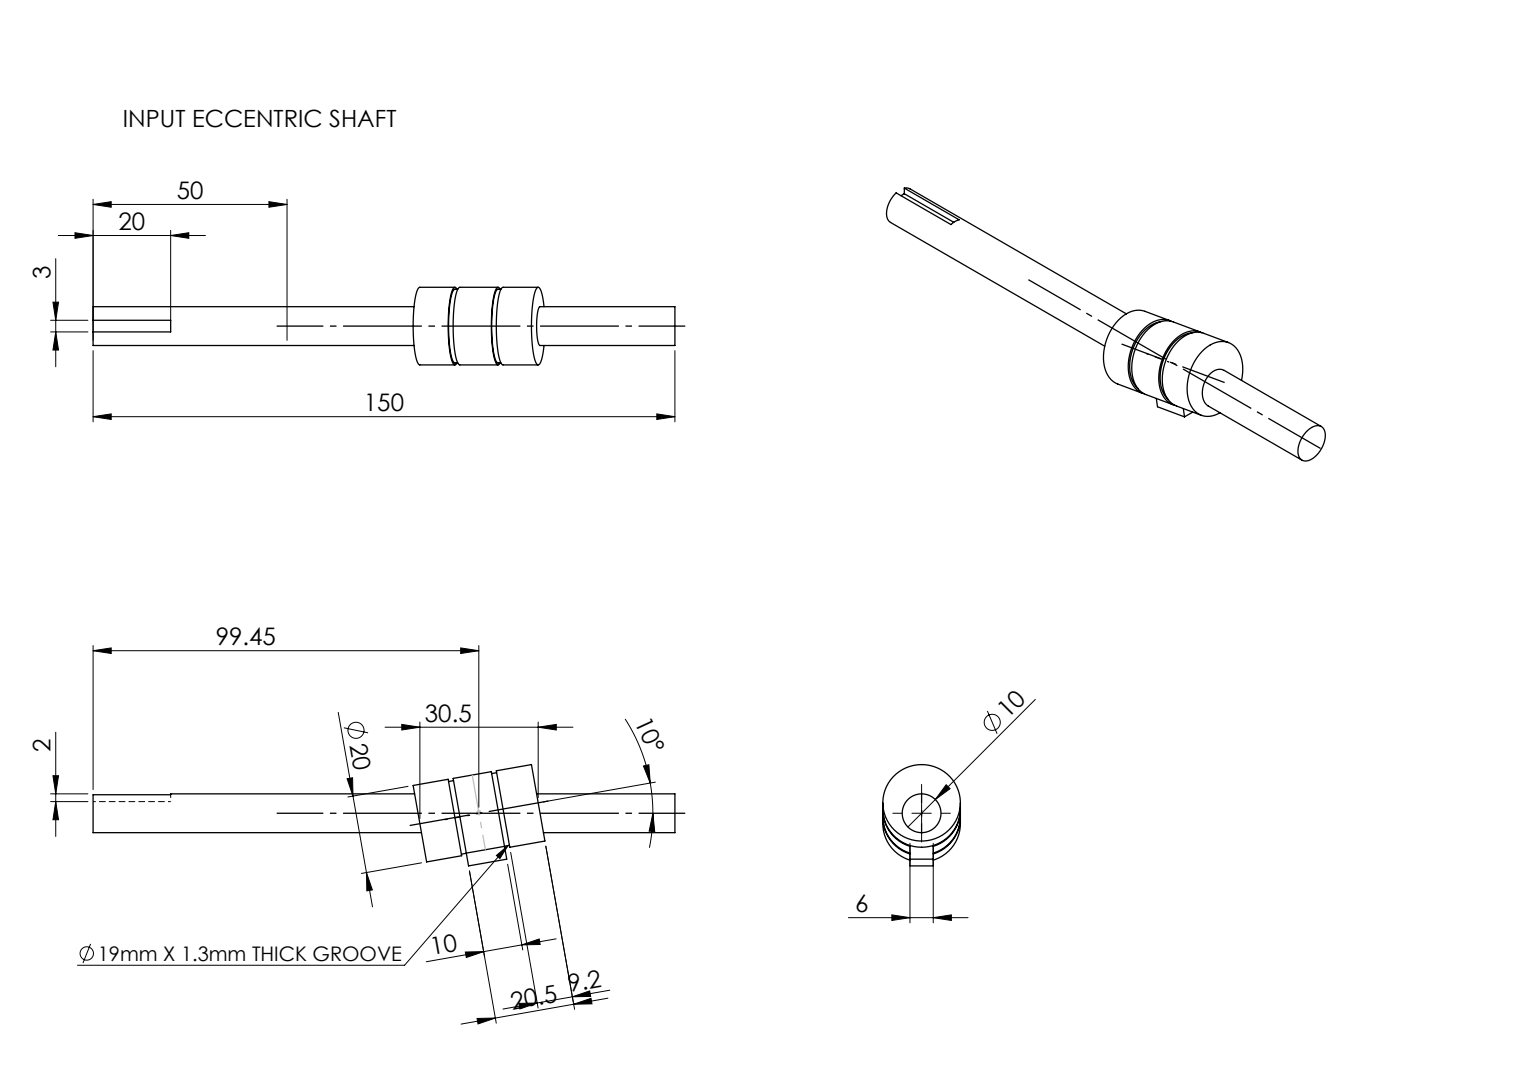
ISO-10303-21;
HEADER;
FILE_DESCRIPTION (('STEP AP214'),
    '1' );
FILE_NAME ('Input Eccentric Shaft.step',
    '2026-10-08T08:02:49',
    ( '' ),
    ( '' ),
    'SwSTEP 2.0',
    'SolidWorks 2026',
    '' );
FILE_SCHEMA (( 'AUTOMOTIVE_DESIGN' ));
ENDSEC;

DATA;
#16=CARTESIAN_POINT ( 'NONE',  ( 16.60577576646022635, -4.999999999999987566, 6.123233995736738672E-16 ) ) ;
#81=ORIENTED_EDGE ( 'NONE', *, *, #43581, .F. ) ;
#144=DIRECTION ( 'NONE',  ( 0.1736481776669314969, -0.9848077530122077983, 5.551115123125780853E-17 ) ) ;
#209=DIRECTION ( 'NONE',  ( -2.280301054154487250E-31, 0.000000000000000000, 1.000000000000000000 ) ) ;
#228=ORIENTED_EDGE ( 'NONE', *, *, #20971, .T. ) ;
#256=EDGE_CURVE ( 'NONE', #600, #12966, #42031, .T. ) ;
#273=FACE_OUTER_BOUND ( 'NONE', #5320, .T. ) ;
#336=MECHANICAL_DESIGN_GEOMETRIC_PRESENTATION_REPRESENTATION('',(#58375),#3336);
#521=AXIS2_PLACEMENT_3D ( 'NONE', #61352, #4959, #18467 ) ;
#546=CARTESIAN_POINT ( 'NONE',  ( 7.147292112312093160, -11.82536368408644911, -2.999999999999993339 ) ) ;
#552=ORIENTED_EDGE ( 'NONE', *, *, #15034, .T. ) ;
#600=VERTEX_POINT ( 'NONE', #1078 ) ;
#662=CARTESIAN_POINT ( 'NONE',  ( -2.700785417809989042, -13.56184546075576769, -3.000000000000003997 ) ) ;
#684=CIRCLE ( 'NONE', #45757, 9.499999999999996447 ) ;
#760=ORIENTED_EDGE ( 'NONE', *, *, #60258, .F. ) ;
#970=FACE_BOUND ( 'NONE', #13663, .T. ) ;
#1006=EDGE_CURVE ( 'NONE', #14410, #28664, #11050, .T. ) ;
#1078=CARTESIAN_POINT ( 'NONE',  ( -79.49999999999975842, 4.769696007084731626, 1.500000000000002220 ) ) ;
#1209=EDGE_CURVE ( 'NONE', #37522, #55939, #6365, .T. ) ;
#1224=CARTESIAN_POINT ( 'NONE',  ( -99.49999999999975842, -9.382821356248120971E-15, -1.500000000000001554 ) ) ;
#1342=LINE ( 'NONE', #2271, #20424 ) ;
#1460=DIRECTION ( 'NONE',  ( -0.1736481776669314137, 0.9848077530122079093, -5.551115123125779004E-17 ) ) ;
#1495=DIRECTION ( 'NONE',  ( -0.1736481776669314137, 0.9848077530122077983, -5.551115123125779004E-17 ) ) ;
#1496=ORIENTED_EDGE ( 'NONE', *, *, #49753, .T. ) ;
#1702=DIRECTION ( 'NONE',  ( 0.1736481776669314969, -0.9848077530122077983, 5.551115123125780853E-17 ) ) ;
#1775=DIRECTION ( 'NONE',  ( -0.9848077530122080203, -0.1736481776669315524, 2.220446049250313574E-16 ) ) ;
#1945=CYLINDRICAL_SURFACE ( 'NONE', #29493, 5.000000000000000000 ) ;
#2107=ORIENTED_EDGE ( 'NONE', *, *, #50234, .F. ) ;
#2130=CARTESIAN_POINT ( 'NONE',  ( -3.282060897439244229, -10.26526840094481052, -2.999999999999990674 ) ) ;
#2158=LINE ( 'NONE', #58242, #51760 ) ;
#2250=FACE_OUTER_BOUND ( 'NONE', #32718, .T. ) ;
#2271=CARTESIAN_POINT ( 'NONE',  ( -49.49999999999975842, -5.000000000000000000, 6.123233995736873765E-16 ) ) ;
#2292=ORIENTED_EDGE ( 'NONE', *, *, #4943, .T. ) ;
#2304=CIRCLE ( 'NONE', #10339, 10.00000000000000000 ) ;
#2335=PLANE ( 'NONE',  #54882 ) ;
#2340=LINE ( 'NONE', #46219, #9470 ) ;
#2383=DIRECTION ( 'NONE',  ( -1.000000000000000000, -1.836970198721027715E-16, 2.218671295934095703E-31 ) ) ;
#2463=CIRCLE ( 'NONE', #33486, 10.00000000000000711 ) ;
#2467=DIRECTION ( 'NONE',  ( 0.9848077530122080203, 0.1736481776669315524, -2.220446049250313574E-16 ) ) ;
#2493=DIRECTION ( 'NONE',  ( 4.437342591868191405E-31, -1.000000000000000000, -4.551914400963141816E-15 ) ) ;
#2607=ORIENTED_EDGE ( 'NONE', *, *, #38979, .F. ) ;
#2638=CARTESIAN_POINT ( 'NONE',  ( 7.147292112312088719, -11.82536368408648286, 3.000000000000017764 ) ) ;
#2691=VERTEX_POINT ( 'NONE', #5356 ) ;
#2704=CARTESIAN_POINT ( 'NONE',  ( -4.923482091946712380, -0.9563062221994939049, 3.000000000000061284 ) ) ;
#2772=ORIENTED_EDGE ( 'NONE', *, *, #49016, .T. ) ;
#2860=PRODUCT_DEFINITION_FORMATION_WITH_SPECIFIED_SOURCE ( 'ANY', '', #16779, .NOT_KNOWN. ) ;
#2948=DIRECTION ( 'NONE',  ( 2.280301054154487250E-31, 0.000000000000000000, -1.000000000000000000 ) ) ;
#3012=EDGE_LOOP ( 'NONE', ( #34469, #21920 ) ) ;
#3051=DIRECTION ( 'NONE',  ( 1.000000000000000000, 1.836970198721027962E-16, -2.033782021272921061E-31 ) ) ;
#3068=ADVANCED_FACE ( 'NONE', ( #57283 ), #53218, .F. ) ;
#3094=ADVANCED_FACE ( 'NONE', ( #273, #23485 ), #33217, .F. ) ;
#3103=EDGE_CURVE ( 'NONE', #36669, #44819, #10148, .T. ) ;
#3198=CIRCLE ( 'NONE', #15257, 5.000000000000000000 ) ;
#3247=ORIENTED_EDGE ( 'NONE', *, *, #59161, .T. ) ;
#3316=SURFACE_STYLE_FILL_AREA ( #40051 ) ;
#3325=VERTEX_POINT ( 'NONE', #34601 ) ;
#3336=( GEOMETRIC_REPRESENTATION_CONTEXT ( 3 ) GLOBAL_UNCERTAINTY_ASSIGNED_CONTEXT ( ( #22977 ) ) GLOBAL_UNIT_ASSIGNED_CONTEXT ( ( #55629, #50939, #7716 ) ) REPRESENTATION_CONTEXT ( 'NONE', 'WORKASPACE' ) );
#3383=DIRECTION ( 'NONE',  ( 0.1736481776669314969, -0.9848077530122079093, -4.496403249731880833E-15 ) ) ;
#3463=ORIENTED_EDGE ( 'NONE', *, *, #44142, .T. ) ;
#3467=CARTESIAN_POINT ( 'NONE',  ( -16.60577576646023701, 5.000000000000008882, -10.00000000000000711 ) ) ;
#3542=VECTOR ( 'NONE', #6303, 1000.000000000000114 ) ;
#3667=EDGE_CURVE ( 'NONE', #55095, #36276, #45940, .T. ) ;
#3711=EDGE_LOOP ( 'NONE', ( #32062, #21018 ) ) ;
#3726=ORIENTED_EDGE ( 'NONE', *, *, #22675, .T. ) ;
#3756=LINE ( 'NONE', #37313, #23956 ) ;
#3759=CARTESIAN_POINT ( 'NONE',  ( 0.000000000000000000, 0.000000000000000000, 0.000000000000000000 ) ) ;
#4057=EDGE_LOOP ( 'NONE', ( #59854, #35436, #34264, #58108, #27155 ) ) ;
#4066=EDGE_CURVE ( 'NONE', #5305, #44819, #39472, .T. ) ;
#4310=VECTOR ( 'NONE', #6048, 1000.000000000000000 ) ;
#4540=CYLINDRICAL_SURFACE ( 'NONE', #31521, 5.000000000000000000 ) ;
#4556=CARTESIAN_POINT ( 'NONE',  ( -6.573139779782565029, 8.399367431416496999, 5.684374357154926636E-14 ) ) ;
#4569=CARTESIAN_POINT ( 'NONE',  ( -16.60577576646023346, 5.000000000000006217, 4.095239503579248533E-30 ) ) ;
#4744=UNCERTAINTY_MEASURE_WITH_UNIT (LENGTH_MEASURE( 1.000000000000000082E-05 ), #37630, 'distance_accuracy_value', 'NONE');
#4762=DIRECTION ( 'NONE',  ( 0.9848077530122080203, 0.1736481776669314692, -5.551115123125783935E-17 ) ) ;
#4915=PLANE ( 'NONE',  #47230 ) ;
#4939=ORIENTED_EDGE ( 'NONE', *, *, #56201, .T. ) ;
#4943=EDGE_CURVE ( 'NONE', #55095, #58934, #3756, .T. ) ;
#4959=DIRECTION ( 'NONE',  ( 0.9848077530122080203, 0.1736481776669314692, -5.551115123125783935E-17 ) ) ;
#4976=DIRECTION ( 'NONE',  ( 0.1736481776669316079, -0.9848077530122079093, -5.551115123125822145E-17 ) ) ;
#5037=DIRECTION ( 'NONE',  ( -0.9848077530122079093, -0.1736481776669316357, -2.245658157333249735E-31 ) ) ;
#5054=DIRECTION ( 'NONE',  ( 0.000000000000000000, -1.000000000000000000, 0.000000000000000000 ) ) ;
#5130=CARTESIAN_POINT ( 'NONE',  ( 6.189768672337906175, 1.091423221261470733, -2.362915713819767774E-16 ) ) ;
#5234=VERTEX_POINT ( 'NONE', #12508 ) ;
#5274=ADVANCED_FACE ( 'NONE', ( #22206 ), #13427, .T. ) ;
#5305=VERTEX_POINT ( 'NONE', #28127 ) ;
#5320=EDGE_LOOP ( 'NONE', ( #35865, #19753 ) ) ;
#5356=CARTESIAN_POINT ( 'NONE',  ( 7.839426360173757047, -8.264250432354510068, 2.910643653149724807E-16 ) ) ;
#5414=DIRECTION ( 'NONE',  ( -0.1736481776669316357, 0.9848077530122079093, -5.551115123125819680E-17 ) ) ;
#5426=CARTESIAN_POINT ( 'NONE',  ( -15.25000000000000711, -2.688986455804108555, -9.952330921218299798E-16 ) ) ;
#5445=DIRECTION ( 'NONE',  ( 0.1736481776669314414, -0.9848077530122079093, 5.551115123125779621E-17 ) ) ;
#5497=EDGE_CURVE ( 'NONE', #2691, #3325, #18968, .T. ) ;
#5596=DIRECTION ( 'NONE',  ( -2.341930812374879235E-31, 1.110223024625156540E-16, 1.000000000000000000 ) ) ;
#5608=EDGE_CURVE ( 'NONE', #6174, #52714, #38324, .T. ) ;
#5613=DIRECTION ( 'NONE',  ( 1.000000000000000000, 1.836970198721029194E-16, -6.779273404243071298E-32 ) ) ;
#5645=DIRECTION ( 'NONE',  ( -2.280301054154487250E-31, 0.000000000000000000, 1.000000000000000000 ) ) ;
#5788=ORIENTED_EDGE ( 'NONE', *, *, #38677, .F. ) ;
#5814=VECTOR ( 'NONE', #17909, 1000.000000000000114 ) ;
#5835=ORIENTED_EDGE ( 'NONE', *, *, #15034, .F. ) ;
#5838=EDGE_CURVE ( 'NONE', #61564, #15021, #37028, .T. ) ;
#5904=CARTESIAN_POINT ( 'NONE',  ( 7.839426360173755270, -8.264250432354510068, 2.910643653149725793E-16 ) ) ;
#5997=EDGE_LOOP ( 'NONE', ( #8432, #36468, #1496, #44361, #29422 ) ) ;
#6020=CARTESIAN_POINT ( 'NONE',  ( 13.51351822333067965, 12.53706398592619209, -3.269553361041724978E-15 ) ) ;
#6048=DIRECTION ( 'NONE',  ( 1.000000000000000000, 1.836970198721027962E-16, -2.033782021272921061E-31 ) ) ;
#6061=ORIENTED_EDGE ( 'NONE', *, *, #8274, .T. ) ;
#6089=FACE_OUTER_BOUND ( 'NONE', #38846, .T. ) ;
#6119=EDGE_CURVE ( 'NONE', #24949, #36033, #38874, .T. ) ;
#6124=CARTESIAN_POINT ( 'NONE',  ( -79.49999999999975842, 5.000000000000006217, -1.500000000000003109 ) ) ;
#6174=VERTEX_POINT ( 'NONE', #36331 ) ;
#6215=CIRCLE ( 'NONE', #55238, 9.500000000000000000 ) ;
#6238=CARTESIAN_POINT ( 'NONE',  ( -4.482327238996802521, -10.94462134745707793, 2.754595595722048466E-16 ) ) ;
#6266=CIRCLE ( 'NONE', #17360, 10.00000000000000711 ) ;
#6303=DIRECTION ( 'NONE',  ( 0.9848077530122079093, 0.1736481776669314414, -5.551115123125783935E-17 ) ) ;
#6320=FACE_OUTER_BOUND ( 'NONE', #15017, .T. ) ;
#6363=EDGE_LOOP ( 'NONE', ( #27773, #60605, #46866, #11752 ) ) ;
#6365=( BOUNDED_CURVE ( )  B_SPLINE_CURVE ( 3, ( #9106, #3467, #14445, #61399 ),
 .UNSPECIFIED., .F., .F. ) 
 B_SPLINE_CURVE_WITH_KNOTS ( ( 4, 4 ),
 ( 3.141592653589793116, 6.283185307179586232 ),
 .UNSPECIFIED. ) 
 CURVE ( )  GEOMETRIC_REPRESENTATION_ITEM ( )  RATIONAL_B_SPLINE_CURVE ( ( 1.000000000000000000, 0.3333333333333333703, 0.3333333333333333703, 1.000000000000000000 ) ) 
 REPRESENTATION_ITEM ( '' )  );
#6400=VECTOR ( 'NONE', #40749, 1000.000000000000114 ) ;
#6421=AXIS2_PLACEMENT_3D ( 'NONE', #54757, #11891, #30970 ) ;
#6556=ORIENTED_EDGE ( 'NONE', *, *, #31470, .T. ) ;
#6626=CIRCLE ( 'NONE', #41706, 10.00000000000000711 ) ;
#6656=CARTESIAN_POINT ( 'NONE',  ( -15.25000000000000711, -2.688986455804108555, -9.952330921218299798E-16 ) ) ;
#6755=ORIENTED_EDGE ( 'NONE', *, *, #47460, .F. ) ;
#6883=DIRECTION ( 'NONE',  ( 0.9848077530122079093, 0.1736481776669314414, -5.551115123125783935E-17 ) ) ;
#6909=LINE ( 'NONE', #59544, #31718 ) ;
#6946=EDGE_LOOP ( 'NONE', ( #22828, #2607, #48957, #16108 ) ) ;
#7136=CARTESIAN_POINT ( 'NONE',  ( -99.49999999999975842, 2.999999999999993339, -1.278713541334263340E-16 ) ) ;
#7167=ORIENTED_EDGE ( 'NONE', *, *, #3667, .T. ) ;
#7246=EDGE_LOOP ( 'NONE', ( #40911, #30741 ) ) ;
#7323=EDGE_CURVE ( 'NONE', #15612, #55623, #24534, .T. ) ;
#7388=EDGE_LOOP ( 'NONE', ( #37494, #6556, #11509, #54224 ) ) ;
#7627=ADVANCED_FACE ( 'NONE', ( #34701, #15596 ), #40653, .F. ) ;
#7716=( NAMED_UNIT ( * ) SI_UNIT ( $, .STERADIAN. ) SOLID_ANGLE_UNIT ( ) );
#7789=VERTEX_POINT ( 'NONE', #60322 ) ;
#7823=AXIS2_PLACEMENT_3D ( 'NONE', #42228, #55976, #37524 ) ;
#7872=EDGE_LOOP ( 'NONE', ( #48131, #29211, #57257, #43270 ) ) ;
#7987=EDGE_CURVE ( 'NONE', #21914, #24949, #48711, .T. ) ;
#8086=DIRECTION ( 'NONE',  ( 0.1736481776669314137, -0.9848077530122077983, 9.436895709313830594E-16 ) ) ;
#8108=CARTESIAN_POINT ( 'NONE',  ( -14.84250595937556483, -4.999999999999993783, 6.123233995736803753E-16 ) ) ;
#8261=FACE_OUTER_BOUND ( 'NONE', #5997, .T. ) ;
#8274=EDGE_CURVE ( 'NONE', #37463, #37711, #43978, .T. ) ;
#8432=ORIENTED_EDGE ( 'NONE', *, *, #41048, .T. ) ;
#8496=DIRECTION ( 'NONE',  ( 0.000000000000000000, 1.000000000000000000, 0.000000000000000000 ) ) ;
#8549=ORIENTED_EDGE ( 'NONE', *, *, #57307, .F. ) ;
#8597=DIRECTION ( 'NONE',  ( 1.000000000000000000, 1.836970198721029194E-16, -6.779273404243071298E-32 ) ) ;
#8794=ORIENTED_EDGE ( 'NONE', *, *, #56127, .F. ) ;
#8921=EDGE_CURVE ( 'NONE', #37463, #45480, #43484, .T. ) ;
#8945=ORIENTED_EDGE ( 'NONE', *, *, #1006, .F. ) ;
#8994=FACE_OUTER_BOUND ( 'NONE', #13159, .T. ) ;
#9097=LINE ( 'NONE', #28206, #17938 ) ;
#9106=CARTESIAN_POINT ( 'NONE',  ( -16.60577576646023346, 5.000000000000006217, 4.095239503579248533E-30 ) ) ;
#9111=CARTESIAN_POINT ( 'NONE',  ( 3.259860905586184021, 10.22135424391044012, 4.719314477116953545E-16 ) ) ;
#9189=ADVANCED_FACE ( 'NONE', ( #2250 ), #1945, .T. ) ;
#9464=ORIENTED_EDGE ( 'NONE', *, *, #59161, .F. ) ;
#9470=VECTOR ( 'NONE', #55576, 1000.000000000000114 ) ;
#9517=DIRECTION ( 'NONE',  ( 0.9848077530122080203, 0.1736481776669315524, -2.220446049250313574E-16 ) ) ;
#9697=CARTESIAN_POINT ( 'NONE',  ( -4.923482091946715045, -0.9563062221994793610, 5.749747411347113621E-14 ) ) ;
#9732=ORIENTED_EDGE ( 'NONE', *, *, #57586, .F. ) ;
#9743=ORIENTED_EDGE ( 'NONE', *, *, #57307, .T. ) ;
#9943=CARTESIAN_POINT ( 'NONE',  ( -79.49999999999975842, -5.510910596163058790E-15, 1.848892746611746419E-29 ) ) ;
#10032=LINE ( 'NONE', #1224, #50554 ) ;
#10040=ORIENTED_EDGE ( 'NONE', *, *, #25957, .F. ) ;
#10148=CIRCLE ( 'NONE', #37175, 9.499999999999996447 ) ;
#10339=AXIS2_PLACEMENT_3D ( 'NONE', #43193, #23755, #42890 ) ;
#10511=VECTOR ( 'NONE', #23069, 1000.000000000000000 ) ;
#10651=CARTESIAN_POINT ( 'NONE',  ( -99.50001199999974233, 5.000000000000003553, -1.500000000000008216 ) ) ;
#10767=DIRECTION ( 'NONE',  ( 1.000000000000000000, 1.836970198721027962E-16, -2.033782021272921061E-31 ) ) ;
#10802=PLANE ( 'NONE',  #13161 ) ;
#10824=CYLINDRICAL_SURFACE ( 'NONE', #48633, 5.000000000000000000 ) ;
#10920=ORIENTED_EDGE ( 'NONE', *, *, #56201, .F. ) ;
#11050=LINE ( 'NONE', #43650, #12094 ) ;
#11308=DIRECTION ( 'NONE',  ( 0.9848077530122079093, 0.1736481776669315802, -5.551115123125782086E-17 ) ) ;
#11337=ORIENTED_EDGE ( 'NONE', *, *, #53081, .F. ) ;
#11483=LINE ( 'NONE', #49377, #28508 ) ;
#11509=ORIENTED_EDGE ( 'NONE', *, *, #17141, .F. ) ;
#11621=VERTEX_POINT ( 'NONE', #13879 ) ;
#11625=CYLINDRICAL_SURFACE ( 'NONE', #47390, 9.500000000000000000 ) ;
#11673=( GEOMETRIC_REPRESENTATION_CONTEXT ( 3 ) GLOBAL_UNCERTAINTY_ASSIGNED_CONTEXT ( ( #4744 ) ) GLOBAL_UNIT_ASSIGNED_CONTEXT ( ( #37630, #51074, #32298 ) ) REPRESENTATION_CONTEXT ( 'NONE', 'WORKASPACE' ) );
#11752=ORIENTED_EDGE ( 'NONE', *, *, #1006, .T. ) ;
#11830=ADVANCED_FACE ( 'NONE', ( #36309 ), #22194, .F. ) ;
#11891=DIRECTION ( 'NONE',  ( 0.9848077530122080203, 0.1736481776669315524, -2.220446049250313574E-16 ) ) ;
#11971=AXIS2_PLACEMENT_3D ( 'NONE', #54925, #31133, #50241 ) ;
#12089=DIRECTION ( 'NONE',  ( -0.1736481776669314137, 0.9848077530122079093, -5.551115123125779004E-17 ) ) ;
#12094=VECTOR ( 'NONE', #48624, 1000.000000000000114 ) ;
#12147=CARTESIAN_POINT ( 'NONE',  ( -6.203732170862584994, -1.182048853166489222, 5.744326400484686099E-14 ) ) ;
#12196=LINE ( 'NONE', #7136, #22678 ) ;
#12222=ORIENTED_EDGE ( 'NONE', *, *, #41831, .T. ) ;
#12249=FACE_OUTER_BOUND ( 'NONE', #6946, .T. ) ;
#12439=LINE ( 'NONE', #2704, #10511 ) ;
#12454=ADVANCED_FACE ( 'NONE', ( #44944 ), #19585, .T. ) ;
#12464=EDGE_LOOP ( 'NONE', ( #16584, #53415 ) ) ;
#12508=CARTESIAN_POINT ( 'NONE',  ( 6.559176281257887098, -8.489993063321520594, 3.632288619156076459E-16 ) ) ;
#12583=DIRECTION ( 'NONE',  ( 0.9848077530122079093, 0.1736481776669315524, -5.551115123125781470E-17 ) ) ;
#12627=CIRCLE ( 'NONE', #32600, 10.00000000000000355 ) ;
#12840=ORIENTED_EDGE ( 'NONE', *, *, #43546, .F. ) ;
#12842=EDGE_CURVE ( 'NONE', #38501, #36669, #6909, .T. ) ;
#12897=SURFACE_STYLE_USAGE ( .BOTH. , #46107 ) ;
#12966=VERTEX_POINT ( 'NONE', #27278 ) ;
#13133=ORIENTED_EDGE ( 'NONE', *, *, #47160, .T. ) ;
#13159=EDGE_LOOP ( 'NONE', ( #46438, #10040, #35648, #40443 ) ) ;
#13161=AXIS2_PLACEMENT_3D ( 'NONE', #58376, #58684, #39316 ) ;
#13350=ORIENTED_EDGE ( 'NONE', *, *, #25260, .T. ) ;
#13403=CARTESIAN_POINT ( 'NONE',  ( -49.49999999999975842, 1.232595164407830946E-29, 1.078520768856852078E-29 ) ) ;
#13427=CYLINDRICAL_SURFACE ( 'NONE', #37981, 10.00000000000000711 ) ;
#13470=AXIS2_PLACEMENT_3D ( 'NONE', #34635, #44665, #1702 ) ;
#13663=EDGE_LOOP ( 'NONE', ( #48253, #13133 ) ) ;
#13690=CIRCLE ( 'NONE', #49659, 10.00000000000000711 ) ;
#13778=CARTESIAN_POINT ( 'NONE',  ( -99.49999999999975842, -5.000000000000009770, 6.123233995736898417E-16 ) ) ;
#13822=DIRECTION ( 'NONE',  ( 1.000000000000000000, 0.000000000000000000, 0.000000000000000000 ) ) ;
#13879=CARTESIAN_POINT ( 'NONE',  ( -3.282060897439242453, -10.26526840094480164, 3.000000000000015987 ) ) ;
#13914=DIRECTION ( 'NONE',  ( -0.1736481776669312471, 0.9848077530122077983, -5.551115123125779621E-17 ) ) ;
#14098=ORIENTED_EDGE ( 'NONE', *, *, #8274, .F. ) ;
#14410=VERTEX_POINT ( 'NONE', #60838 ) ;
#14445=CARTESIAN_POINT ( 'NONE',  ( -14.84250595937557549, -4.999999999999997335, -10.00000000000000711 ) ) ;
#14662=DIRECTION ( 'NONE',  ( -0.9848077530122079093, -0.1736481776669316079, 5.551115123125783935E-17 ) ) ;
#14677=AXIS2_PLACEMENT_3D ( 'NONE', #3759, #61387, #13822 ) ;
#14867=EDGE_CURVE ( 'NONE', #37711, #37128, #6626, .T. ) ;
#15017=EDGE_LOOP ( 'NONE', ( #23318, #49149 ) ) ;
#15021=VERTEX_POINT ( 'NONE', #2130 ) ;
#15034=EDGE_CURVE ( 'NONE', #35339, #16043, #12196, .T. ) ;
#15131=CARTESIAN_POINT ( 'NONE',  ( -4.923482091946717709, -0.9563062221994661494, -2.999999999999945377 ) ) ;
#15141=FACE_OUTER_BOUND ( 'NONE', #37722, .T. ) ;
#15166=AXIS2_PLACEMENT_3D ( 'NONE', #42617, #61677, #47614 ) ;
#15257=AXIS2_PLACEMENT_3D ( 'NONE', #41389, #55135, #44857 ) ;
#15277=DIRECTION ( 'NONE',  ( -0.9848077530122079093, -0.1736481776669316357, -2.245658157333249735E-31 ) ) ;
#15460=DIRECTION ( 'NONE',  ( 1.000000000000000000, 1.836970198721027715E-16, -2.218671295934095703E-31 ) ) ;
#15567=DIRECTION ( 'NONE',  ( 1.836970198721031906E-16, -1.000000000000000000, 1.110223024625156540E-16 ) ) ;
#15596=FACE_OUTER_BOUND ( 'NONE', #3711, .T. ) ;
#15612=VERTEX_POINT ( 'NONE', #37792 ) ;
#15683=ADVANCED_FACE ( 'NONE', ( #44335 ), #10802, .T. ) ;
#15707=( GEOMETRIC_REPRESENTATION_CONTEXT ( 3 ) GLOBAL_UNCERTAINTY_ASSIGNED_CONTEXT ( ( #28578 ) ) GLOBAL_UNIT_ASSIGNED_CONTEXT ( ( #40801, #36092, #26980 ) ) REPRESENTATION_CONTEXT ( 'NONE', 'WORKASPACE' ) );
#15771=DIRECTION ( 'NONE',  ( -0.9848077530122079093, -0.1736481776669315802, 1.387778780781445367E-17 ) ) ;
#15843=PLANE ( 'NONE',  #57644 ) ;
#15894=LINE ( 'NONE', #25582, #26913 ) ;
#16043=VERTEX_POINT ( 'NONE', #31288 ) ;
#16108=ORIENTED_EDGE ( 'NONE', *, *, #3103, .T. ) ;
#16222=LINE ( 'NONE', #19693, #35442 ) ;
#16226=ADVANCED_FACE ( 'NONE', ( #19984, #39098 ), #4915, .T. ) ;
#16257=DIRECTION ( 'NONE',  ( -2.280301054154487250E-31, 0.000000000000000000, 1.000000000000000000 ) ) ;
#16372=DIRECTION ( 'NONE',  ( 1.000000000000000000, 1.836970198721027962E-16, -2.033782021272921061E-31 ) ) ;
#16416=ORIENTED_EDGE ( 'NONE', *, *, #5497, .F. ) ;
#16584=ORIENTED_EDGE ( 'NONE', *, *, #37344, .T. ) ;
#16779=PRODUCT ( 'Input Eccentric Shaft', 'Input Eccentric Shaft', '', ( #21797 ) ) ;
#16838=FILL_AREA_STYLE_COLOUR ( '', #26379 ) ;
#16911=VECTOR ( 'NONE', #10767, 1000.000000000000000 ) ;
#16928=AXIS2_PLACEMENT_3D ( 'NONE', #43300, #5037, #5645 ) ;
#16977=EDGE_LOOP ( 'NONE', ( #16416, #21342 ) ) ;
#17137=EDGE_CURVE ( 'NONE', #51465, #6174, #57525, .T. ) ;
#17141=EDGE_CURVE ( 'NONE', #5234, #46104, #6215, .T. ) ;
#17186=DIRECTION ( 'NONE',  ( 0.1736481776669316079, -0.9848077530122079093, -5.551115123125822145E-17 ) ) ;
#17360=AXIS2_PLACEMENT_3D ( 'NONE', #6656, #27040, #35840 ) ;
#17530=AXIS2_PLACEMENT_3D ( 'NONE', #53533, #58538, #33538 ) ;
#17550=ORIENTED_EDGE ( 'NONE', *, *, #256, .T. ) ;
#17661=CARTESIAN_POINT ( 'NONE',  ( 6.189768672337906175, 1.091423221261470733, -2.362915713819767774E-16 ) ) ;
#17747=CIRCLE ( 'NONE', #31747, 9.500000000000000000 ) ;
#17909=DIRECTION ( 'NONE',  ( -0.9848077530122079093, -0.1736481776669314414, 5.551115123125783935E-17 ) ) ;
#17938=VECTOR ( 'NONE', #47322, 1000.000000000000000 ) ;
#18111=DIRECTION ( 'NONE',  ( 0.9848077530122080203, 0.1736481776669315524, -2.220446049250313574E-16 ) ) ;
#18143=ORIENTED_EDGE ( 'NONE', *, *, #29937, .T. ) ;
#18202=SHAPE_REPRESENTATION_RELATIONSHIP ( 'NONE' , 'NONE' ,  #27649, #51224 ) ;
#18205=CARTESIAN_POINT ( 'NONE',  ( -79.49999999999975842, 4.999999999999996447, 1.500000000000000444 ) ) ;
#18371=EDGE_LOOP ( 'NONE', ( #14098, #56883, #20608, #20746 ) ) ;
#18437=LINE ( 'NONE', #23134, #21997 ) ;
#18467=DIRECTION ( 'NONE',  ( -0.1736481776669312471, 0.9848077530122077983, -5.551115123125779621E-17 ) ) ;
#18610=VECTOR ( 'NONE', #39599, 1000.000000000000000 ) ;
#18652=EDGE_LOOP ( 'NONE', ( #48864, #5788 ) ) ;
#18852=CARTESIAN_POINT ( 'NONE',  ( 14.84250595937556660, 5.000000000000015099, 10.00000000000000711 ) ) ;
#18878=DIRECTION ( 'NONE',  ( -0.1736481776669316357, 0.9848077530122079093, 4.662936703425656681E-15 ) ) ;
#18968=CIRCLE ( 'NONE', #20962, 9.500000000000000000 ) ;
#19051=EDGE_LOOP ( 'NONE', ( #52943, #17550, #37320, #4939 ) ) ;
#19487=FACE_OUTER_BOUND ( 'NONE', #29462, .T. ) ;
#19523=FACE_OUTER_BOUND ( 'NONE', #27402, .T. ) ;
#19585=CYLINDRICAL_SURFACE ( 'NONE', #21802, 9.500000000000005329 ) ;
#19614=ORIENTED_EDGE ( 'NONE', *, *, #5838, .T. ) ;
#19665=CARTESIAN_POINT ( 'NONE',  ( 4.540110984502055302, 10.44709687487745065, 3.997669511110601399E-16 ) ) ;
#19693=CARTESIAN_POINT ( 'NONE',  ( 4.924595438175360940, 0.7801755544698492084, -2.999999999999945821 ) ) ;
#19729=DIRECTION ( 'NONE',  ( -2.341930812374879235E-31, 1.110223024625156540E-16, 1.000000000000000000 ) ) ;
#19753=ORIENTED_EDGE ( 'NONE', *, *, #20975, .T. ) ;
#19815=AXIS2_PLACEMENT_3D ( 'NONE', #22245, #28781, #61657 ) ;
#19921=PRODUCT_DEFINITION_SHAPE ( 'NONE', 'NONE',  #43635 ) ;
#19984=FACE_OUTER_BOUND ( 'NONE', #39897, .T. ) ;
#20216=CIRCLE ( 'NONE', #45267, 9.500000000000000000 ) ;
#20360=CARTESIAN_POINT ( 'NONE',  ( -2.700785417809989042, -13.56184546075576769, -3.000000000000003997 ) ) ;
#20424=VECTOR ( 'NONE', #20479, 1000.000000000000000 ) ;
#20479=DIRECTION ( 'NONE',  ( 1.000000000000000000, 1.836970198721027962E-16, -2.033782021272921061E-31 ) ) ;
#20608=ORIENTED_EDGE ( 'NONE', *, *, #57586, .T. ) ;
#20692=PLANE ( 'NONE',  #32932 ) ;
#20746=ORIENTED_EDGE ( 'NONE', *, *, #14867, .F. ) ;
#20789=CIRCLE ( 'NONE', #19815, 5.000000000000000000 ) ;
#20962=AXIS2_PLACEMENT_3D ( 'NONE', #17661, #51456, #27058 ) ;
#20971=EDGE_CURVE ( 'NONE', #24192, #11621, #2463, .T. ) ;
#20975=EDGE_CURVE ( 'NONE', #36033, #24949, #47475, .T. ) ;
#21018=ORIENTED_EDGE ( 'NONE', *, *, #22675, .F. ) ;
#21022=VECTOR ( 'NONE', #56389, 1000.000000000000000 ) ;
#21086=CARTESIAN_POINT ( 'NONE',  ( -99.49999999999975842, -9.057560704502469641E-15, 1.500000000000000888 ) ) ;
#21342=ORIENTED_EDGE ( 'NONE', *, *, #30352, .F. ) ;
#21797=PRODUCT_CONTEXT ( 'NONE', #44793, 'mechanical' ) ;
#21802=AXIS2_PLACEMENT_3D ( 'NONE', #53072, #48383, #5445 ) ;
#21914=VERTEX_POINT ( 'NONE', #39550 ) ;
#21920=ORIENTED_EDGE ( 'NONE', *, *, #17137, .T. ) ;
#21942=LINE ( 'NONE', #41080, #56942 ) ;
#21997=VECTOR ( 'NONE', #3383, 1000.000000000000000 ) ;
#22001=ORIENTED_EDGE ( 'NONE', *, *, #53081, .T. ) ;
#22083=FACE_OUTER_BOUND ( 'NONE', #12464, .T. ) ;
#22179=EDGE_CURVE ( 'NONE', #2691, #5234, #33851, .T. ) ;
#22194=PLANE ( 'NONE',  #50757 ) ;
#22206=FACE_OUTER_BOUND ( 'NONE', #33124, .T. ) ;
#22236=CARTESIAN_POINT ( 'NONE',  ( 6.566016632731837888, -8.528786624275497275, -2.999999999999986677 ) ) ;
#22245=CARTESIAN_POINT ( 'NONE',  ( -99.49999999999975842, -9.184850993605117179E-15, 3.081487911019577365E-29 ) ) ;
#22527=CARTESIAN_POINT ( 'NONE',  ( -14.84250595937557016, -4.999999999999995559, 10.00000000000000711 ) ) ;
#22583=AXIS2_PLACEMENT_3D ( 'NONE', #47715, #4762, #13914 ) ;
#22591=FILL_AREA_STYLE ('',( #27590 ) ) ;
#22675=EDGE_CURVE ( 'NONE', #44582, #21914, #25945, .T. ) ;
#22678=VECTOR ( 'NONE', #16257, 1000.000000000000000 ) ;
#22828=ORIENTED_EDGE ( 'NONE', *, *, #4066, .F. ) ;
#22895=ORIENTED_EDGE ( 'NONE', *, *, #38677, .T. ) ;
#22977=UNCERTAINTY_MEASURE_WITH_UNIT (LENGTH_MEASURE( 1.000000000000000082E-05 ), #55629, 'distance_accuracy_value', 'NONE');
#23069=DIRECTION ( 'NONE',  ( 0.1736481776669314969, -0.9848077530122079093, -4.496403249731880833E-15 ) ) ;
#23134=CARTESIAN_POINT ( 'NONE',  ( 4.924595438175366269, 0.7801755544698232292, 3.000000000000058620 ) ) ;
#23309=CARTESIAN_POINT ( 'NONE',  ( -79.49999999999975842, -1.460391307983213802E-14, 1.540743955509788682E-30 ) ) ;
#23313=VECTOR ( 'NONE', #23816, 1000.000000000000114 ) ;
#23318=ORIENTED_EDGE ( 'NONE', *, *, #59797, .F. ) ;
#23485=FACE_BOUND ( 'NONE', #52507, .T. ) ;
#23556=CARTESIAN_POINT ( 'NONE',  ( -15.25000000000000711, -2.688986455804108555, -9.952330921218299798E-16 ) ) ;
#23585=ORIENTED_EDGE ( 'NONE', *, *, #43586, .T. ) ;
#23621=LINE ( 'NONE', #48353, #27892 ) ;
#23676=CARTESIAN_POINT ( 'NONE',  ( -49.49999999999975842, 1.232595164407830946E-29, 1.078520768856852078E-29 ) ) ;
#23755=DIRECTION ( 'NONE',  ( 0.9848077530122077983, 0.1736481776669316079, -1.387778780781445367E-17 ) ) ;
#23816=DIRECTION ( 'NONE',  ( -0.9848077530122079093, -0.1736481776669316079, 5.551115123125783935E-17 ) ) ;
#23872=DIRECTION ( 'NONE',  ( 0.9848077530122080203, 0.1736481776669314692, -5.551115123125783935E-17 ) ) ;
#23896=ORIENTED_EDGE ( 'NONE', *, *, #44390, .T. ) ;
#23956=VECTOR ( 'NONE', #31993, 1000.000000000000000 ) ;
#24192=VERTEX_POINT ( 'NONE', #40694 ) ;
#24450=CARTESIAN_POINT ( 'NONE',  ( 14.84250595937556483, 5.000000000000012434, -2.300655493813809945E-30 ) ) ;
#24534=CIRCLE ( 'NONE', #57551, 10.00000000000000000 ) ;
#24549=CIRCLE ( 'NONE', #37589, 10.00000000000000711 ) ;
#24552=DIRECTION ( 'NONE',  ( 0.1736481776669314137, -0.9848077530122077983, 5.551115123125779004E-17 ) ) ;
#24652=LINE ( 'NONE', #6124, #45372 ) ;
#24742=FACE_OUTER_BOUND ( 'NONE', #56323, .T. ) ;
#24805=VERTEX_POINT ( 'NONE', #29871 ) ;
#24815=PRODUCT_DEFINITION_CONTEXT ( 'detailed design', #50787, 'design' ) ;
#24874=FACE_OUTER_BOUND ( 'NONE', #49710, .T. ) ;
#24909=CIRCLE ( 'NONE', #40942, 5.000000000000000000 ) ;
#24949=VERTEX_POINT ( 'NONE', #37370 ) ;
#25042=VECTOR ( 'NONE', #55448, 1000.000000000000000 ) ;
#25051=FACE_OUTER_BOUND ( 'NONE', #51644, .T. ) ;
#25149=FACE_BOUND ( 'NONE', #16977, .T. ) ;
#25184=CARTESIAN_POINT ( 'NONE',  ( -49.49999999999975842, 5.000000000000000000, 1.078520768856852078E-29 ) ) ;
#25260=EDGE_CURVE ( 'NONE', #36276, #55939, #45783, .T. ) ;
#25365=ORIENTED_EDGE ( 'NONE', *, *, #31470, .F. ) ;
#25513=ORIENTED_EDGE ( 'NONE', *, *, #46681, .T. ) ;
#25582=CARTESIAN_POINT ( 'NONE',  ( 7.147292112312093160, -11.82536368408644911, -2.999999999999993339 ) ) ;
#25609=ORIENTED_EDGE ( 'NONE', *, *, #33336, .T. ) ;
#25711=DIRECTION ( 'NONE',  ( -0.1736481776669316357, 0.9848077530122079093, -5.551115123125819680E-17 ) ) ;
#25744=AXIS2_PLACEMENT_3D ( 'NONE', #9943, #61908, #52216 ) ;
#25790=AXIS2_PLACEMENT_3D ( 'NONE', #30396, #54498, #44234 ) ;
#25791=CYLINDRICAL_SURFACE ( 'NONE', #51920, 10.00000000000000711 ) ;
#25844=DIRECTION ( 'NONE',  ( 1.836970198721033632E-16, -1.000000000000000000, 0.000000000000000000 ) ) ;
#25945=CIRCLE ( 'NONE', #11971, 10.00000000000000711 ) ;
#25957=EDGE_CURVE ( 'NONE', #6174, #51465, #46220, .T. ) ;
#26200=CARTESIAN_POINT ( 'NONE',  ( -79.49999999999975842, -5.510910596163058790E-15, 1.848892746611746419E-29 ) ) ;
#26206=DIRECTION ( 'NONE',  ( 0.9848077530122079093, 0.1736481776669314137, -2.220446049250313081E-16 ) ) ;
#26236=CARTESIAN_POINT ( 'NONE',  ( -14.84250595937556483, -4.999999999999993783, 6.123233995736803753E-16 ) ) ;
#26379=COLOUR_RGB ( '', 0.40784314, 0.44705882, 0.49803922) ;
#26519=CARTESIAN_POINT ( 'NONE',  ( -15.25000000000000711, -2.688986455804108555, -9.952330921218299798E-16 ) ) ;
#26588=ADVANCED_FACE ( 'NONE', ( #53042 ), #37435, .T. ) ;
#26685=CIRCLE ( 'NONE', #32692, 5.000000000000000000 ) ;
#26801=( BOUNDED_CURVE ( )  B_SPLINE_CURVE ( 3, ( #8108, #22527, #33168, #27220 ),
 .UNSPECIFIED., .F., .F. ) 
 B_SPLINE_CURVE_WITH_KNOTS ( ( 4, 4 ),
 ( 0.000000000000000000, 3.141592653589793116 ),
 .UNSPECIFIED. ) 
 CURVE ( )  GEOMETRIC_REPRESENTATION_ITEM ( )  RATIONAL_B_SPLINE_CURVE ( ( 1.000000000000000000, 0.3333333333333333703, 0.3333333333333333703, 1.000000000000000000 ) ) 
 REPRESENTATION_ITEM ( '' )  );
#26913=VECTOR ( 'NONE', #35628, 1000.000000000000000 ) ;
#26949=CARTESIAN_POINT ( 'NONE',  ( -79.49999999999975842, 4.999999999999994671, 1.229372086083732569E-29 ) ) ;
#26980=( NAMED_UNIT ( * ) SI_UNIT ( $, .STERADIAN. ) SOLID_ANGLE_UNIT ( ) );
#27040=DIRECTION ( 'NONE',  ( 0.9848077530122080203, 0.1736481776669315247, -2.220446049250313081E-16 ) ) ;
#27058=DIRECTION ( 'NONE',  ( 0.1736481776669315247, -0.9848077530122079093, 5.551115123125782702E-17 ) ) ;
#27099=ADVANCED_FACE ( 'NONE', ( #50969 ), #36590, .T. ) ;
#27155=ORIENTED_EDGE ( 'NONE', *, *, #45156, .T. ) ;
#27202=ORIENTED_EDGE ( 'NONE', *, *, #41831, .F. ) ;
#27220=CARTESIAN_POINT ( 'NONE',  ( -16.60577576646023346, 5.000000000000006217, 4.095239503579248533E-30 ) ) ;
#27278=CARTESIAN_POINT ( 'NONE',  ( -79.49999999999975842, 2.999999999999996891, 1.500000000000000000 ) ) ;
#27285=CARTESIAN_POINT ( 'NONE',  ( -79.49999999999975842, 4.769696007084728961, -1.500000000000002887 ) ) ;
#27299=ORIENTED_EDGE ( 'NONE', *, *, #5608, .F. ) ;
#27402=EDGE_LOOP ( 'NONE', ( #28240, #228, #47775, #54695 ) ) ;
#27495=DIRECTION ( 'NONE',  ( 0.1736481776669315247, -0.9848077530122079093, 5.551115123125782702E-17 ) ) ;
#27499=CARTESIAN_POINT ( 'NONE',  ( -4.938558936750251149, -0.8708011863679817610, 8.896908036367455278E-17 ) ) ;
#27556=CYLINDRICAL_SURFACE ( 'NONE', #521, 10.00000000000000711 ) ;
#27590=FILL_AREA_STYLE_COLOUR ( '', #50682 ) ;
#27649=SHAPE_REPRESENTATION ( 'Input Eccentric Shaft', ( #14677 ), #15707 ) ;
#27725=LINE ( 'NONE', #52132, #30832 ) ;
#27759=VECTOR ( 'NONE', #47424, 1000.000000000000000 ) ;
#27773=ORIENTED_EDGE ( 'NONE', *, *, #45156, .F. ) ;
#27849=CIRCLE ( 'NONE', #25744, 5.000000000000000000 ) ;
#27857=EDGE_LOOP ( 'NONE', ( #552, #2772, #25513, #27202 ) ) ;
#27866=ADVANCED_FACE ( 'NONE', ( #19487 ), #28252, .F. ) ;
#27892=VECTOR ( 'NONE', #53341, 1000.000000000000114 ) ;
#28102=CYLINDRICAL_SURFACE ( 'NONE', #36371, 5.000000000000000000 ) ;
#28127=CARTESIAN_POINT ( 'NONE',  ( -4.554074483026735898, -10.53772250678246358, 5.913403440073379425E-14 ) ) ;
#28206=CARTESIAN_POINT ( 'NONE',  ( -2.700785417809989042, -13.56184546075576769, -3.000000000000003997 ) ) ;
#28240=ORIENTED_EDGE ( 'NONE', *, *, #44142, .F. ) ;
#28252=PLANE ( 'NONE',  #38892 ) ;
#28254=DIRECTION ( 'NONE',  ( -0.1736481776669312471, 0.9848077530122077983, -5.551115123125779621E-17 ) ) ;
#28434=ORIENTED_EDGE ( 'NONE', *, *, #30352, .T. ) ;
#28473=AXIS2_PLACEMENT_3D ( 'NONE', #41617, #32214, #17186 ) ;
#28508=VECTOR ( 'NONE', #44108, 1000.000000000000114 ) ;
#28578=UNCERTAINTY_MEASURE_WITH_UNIT (LENGTH_MEASURE( 1.000000000000000082E-05 ), #40801, 'distance_accuracy_value', 'NONE');
#28609=LINE ( 'NONE', #33342, #27759 ) ;
#28664=VERTEX_POINT ( 'NONE', #2638 ) ;
#28781=DIRECTION ( 'NONE',  ( -1.000000000000000000, -1.836970198721027715E-16, 2.218671295934095703E-31 ) ) ;
#28821=ADVANCED_FACE ( 'NONE', ( #44834 ), #20692, .T. ) ;
#28928=DIRECTION ( 'NONE',  ( 0.1736481776669315802, -0.9848077530122079093, 5.551115123125782702E-17 ) ) ;
#28929=ADVANCED_FACE ( 'NONE', ( #43930, #970 ), #33584, .F. ) ;
#29164=CARTESIAN_POINT ( 'NONE',  ( 6.566016632682842413, -8.528786624275486616, 3.000000000000020872 ) ) ;
#29211=ORIENTED_EDGE ( 'NONE', *, *, #43546, .T. ) ;
#29418=CARTESIAN_POINT ( 'NONE',  ( -99.50001199999974233, 5.000000000000001776, 1.500000000000000222 ) ) ;
#29422=ORIENTED_EDGE ( 'NONE', *, *, #256, .F. ) ;
#29462=EDGE_LOOP ( 'NONE', ( #23896, #8945, #34005, #22001 ) ) ;
#29493=AXIS2_PLACEMENT_3D ( 'NONE', #59265, #16372, #8496 ) ;
#29559=ADVANCED_FACE ( 'NONE', ( #24874 ), #25791, .T. ) ;
#29739=PLANE ( 'NONE',  #46560 ) ;
#29749=CARTESIAN_POINT ( 'NONE',  ( -7.853389858698435866, 8.173624800449486472, 5.691590806814991163E-14 ) ) ;
#29826=DIRECTION ( 'NONE',  ( 0.1736481776669314969, -0.9848077530122079093, -4.496403249731880833E-15 ) ) ;
#29871=CARTESIAN_POINT ( 'NONE',  ( -99.49999999999975842, 4.769696007084727185, 1.499999999999998446 ) ) ;
#29896=VECTOR ( 'NONE', #58220, 1000.000000000000000 ) ;
#29937=EDGE_CURVE ( 'NONE', #7789, #52714, #3198, .T. ) ;
#30038=CARTESIAN_POINT ( 'NONE',  ( 15.24999999999999289, 2.688986455804112996, 8.896908036367455278E-17 ) ) ;
#30186=LINE ( 'NONE', #25184, #4310 ) ;
#30228=DIRECTION ( 'NONE',  ( -1.000000000000000000, -1.836970198721033632E-16, 2.218671295934095703E-31 ) ) ;
#30352=EDGE_CURVE ( 'NONE', #3325, #2691, #20216, .T. ) ;
#30396=CARTESIAN_POINT ( 'NONE',  ( -4.923482091946715045, -0.9563062221994793610, 5.749747411347113621E-14 ) ) ;
#30464=LINE ( 'NONE', #21086, #18610 ) ;
#30472=DIRECTION ( 'NONE',  ( 0.9848077530122080203, 0.1736481776669314692, -5.551115123125783935E-17 ) ) ;
#30654=MECHANICAL_DESIGN_GEOMETRIC_PRESENTATION_REPRESENTATION('',(#49663),#11673);
#30741=ORIENTED_EDGE ( 'NONE', *, *, #48278, .F. ) ;
#30832=VECTOR ( 'NONE', #8597, 1000.000000000000000 ) ;
#30938=CARTESIAN_POINT ( 'NONE',  ( 14.84250595937556483, 5.000000000000015099, -10.00000000000000711 ) ) ;
#30970=DIRECTION ( 'NONE',  ( 0.1736481776669314137, -0.9848077530122077983, 5.551115123125779621E-17 ) ) ;
#31133=DIRECTION ( 'NONE',  ( 0.9848077530122080203, 0.1736481776669315247, -2.220446049250313081E-16 ) ) ;
#31245=CARTESIAN_POINT ( 'NONE',  ( 16.60577576646022635, -4.999999999999987566, 6.123233995736738672E-16 ) ) ;
#31288=CARTESIAN_POINT ( 'NONE',  ( -99.49999999999975842, 2.999999999999994671, 1.500000000000001554 ) ) ;
#31470=EDGE_CURVE ( 'NONE', #3325, #46104, #48460, .T. ) ;
#31517=CIRCLE ( 'NONE', #28473, 9.499999999999996447 ) ;
#31521=AXIS2_PLACEMENT_3D ( 'NONE', #23676, #33401, #52478 ) ;
#31624=LINE ( 'NONE', #60120, #6400 ) ;
#31718=VECTOR ( 'NONE', #12583, 1000.000000000000000 ) ;
#31747=AXIS2_PLACEMENT_3D ( 'NONE', #34492, #54175, #43917 ) ;
#31993=DIRECTION ( 'NONE',  ( 1.000000000000000000, 1.836970198721027962E-16, -2.033782021272921061E-31 ) ) ;
#32062=ORIENTED_EDGE ( 'NONE', *, *, #50356, .F. ) ;
#32214=DIRECTION ( 'NONE',  ( -0.9848077530122080203, -0.1736481776669315524, 2.220446049250313574E-16 ) ) ;
#32266=ADVANCED_FACE ( 'NONE', ( #12249 ), #11625, .T. ) ;
#32298=( NAMED_UNIT ( * ) SI_UNIT ( $, .STERADIAN. ) SOLID_ANGLE_UNIT ( ) );
#32370=ORIENTED_EDGE ( 'NONE', *, *, #4943, .F. ) ;
#32441=VERTEX_POINT ( 'NONE', #26949 ) ;
#32535=CARTESIAN_POINT ( 'NONE',  ( -15.25000000000000711, -2.688986455804108555, -9.952330921218299798E-16 ) ) ;
#32600=AXIS2_PLACEMENT_3D ( 'NONE', #47483, #43107, #144 ) ;
#32692=AXIS2_PLACEMENT_3D ( 'NONE', #26200, #2383, #59397 ) ;
#32718=EDGE_LOOP ( 'NONE', ( #45990, #25609, #52166, #27299 ) ) ;
#32727=DIRECTION ( 'NONE',  ( 0.9848077530122079093, 0.1736481776669315802, -5.551115123125782086E-17 ) ) ;
#32800=ORIENTED_EDGE ( 'NONE', *, *, #25260, .F. ) ;
#32818=ADVANCED_FACE ( 'NONE', ( #8994 ), #28102, .T. ) ;
#32932=AXIS2_PLACEMENT_3D ( 'NONE', #40755, #39831, #2493 ) ;
#33046=CARTESIAN_POINT ( 'NONE',  ( -4.938558936750251149, -0.8708011863679817610, 8.896908036367455278E-17 ) ) ;
#33124=EDGE_LOOP ( 'NONE', ( #58141, #3463, #61395, #19614 ) ) ;
#33168=CARTESIAN_POINT ( 'NONE',  ( -16.60577576646022990, 5.000000000000008882, 10.00000000000000711 ) ) ;
#33217=PLANE ( 'NONE',  #15166 ) ;
#33259=DIRECTION ( 'NONE',  ( 0.1736481776669315247, -0.9848077530122079093, 5.551115123125782702E-17 ) ) ;
#33336=EDGE_CURVE ( 'NONE', #51465, #7789, #1342, .T. ) ;
#33342=CARTESIAN_POINT ( 'NONE',  ( -79.49999999999975842, 2.999999999999996891, 1.500000000000000000 ) ) ;
#33401=DIRECTION ( 'NONE',  ( 1.000000000000000000, 1.836970198721027962E-16, -2.033782021272921061E-31 ) ) ;
#33486=AXIS2_PLACEMENT_3D ( 'NONE', #27499, #18111, #8086 ) ;
#33538=DIRECTION ( 'NONE',  ( 4.437342591868191405E-31, -1.000000000000000000, -4.551914400963141816E-15 ) ) ;
#33559=ADVANCED_FACE ( 'NONE', ( #52358 ), #42383, .T. ) ;
#33584=PLANE ( 'NONE',  #16928 ) ;
#33838=DIRECTION ( 'NONE',  ( 2.218671295934095703E-31, -1.000000000000000000, 1.110223024625156540E-16 ) ) ;
#33851=LINE ( 'NONE', #5904, #23313 ) ;
#33955=CARTESIAN_POINT ( 'NONE',  ( -99.49999999999975842, 4.769696007084730738, -1.500000000000008438 ) ) ;
#33979=DIRECTION ( 'NONE',  ( -0.1736481776669312471, 0.9848077530122077983, -5.551115123125779621E-17 ) ) ;
#34005=ORIENTED_EDGE ( 'NONE', *, *, #44839, .F. ) ;
#34179=CARTESIAN_POINT ( 'NONE',  ( 16.60577576646022990, -4.999999999999989342, 10.00000000000000711 ) ) ;
#34248=CYLINDRICAL_SURFACE ( 'NONE', #49616, 10.00000000000000711 ) ;
#34264=ORIENTED_EDGE ( 'NONE', *, *, #50707, .T. ) ;
#34266=CARTESIAN_POINT ( 'NONE',  ( -49.49999999999975842, 4.769696007084739620, 1.500000000000005329 ) ) ;
#34469=ORIENTED_EDGE ( 'NONE', *, *, #25957, .T. ) ;
#34492=CARTESIAN_POINT ( 'NONE',  ( 4.909518593422035337, 0.8656805902944597619, 8.896908036367455278E-17 ) ) ;
#34601=CARTESIAN_POINT ( 'NONE',  ( 4.540110984502054414, 10.44709687487745065, 3.997669511110601399E-16 ) ) ;
#34635=CARTESIAN_POINT ( 'NONE',  ( 6.189768672335216770, 1.091423221276722755, -1.945113688487589062E-17 ) ) ;
#34701=FACE_BOUND ( 'NONE', #18652, .T. ) ;
#34739=CARTESIAN_POINT ( 'NONE',  ( 15.24999999999999289, 2.688986455804112996, 8.896908036367455278E-17 ) ) ;
#34957=CARTESIAN_POINT ( 'NONE',  ( -99.49999999999975842, -9.184850993605117179E-15, 3.081487911019577365E-29 ) ) ;
#35339=VERTEX_POINT ( 'NONE', #39739 ) ;
#35436=ORIENTED_EDGE ( 'NONE', *, *, #51896, .F. ) ;
#35442=VECTOR ( 'NONE', #40064, 1000.000000000000000 ) ;
#35628=DIRECTION ( 'NONE',  ( 8.032841876251139751E-16, -4.551914400963141816E-15, 1.000000000000000000 ) ) ;
#35648=ORIENTED_EDGE ( 'NONE', *, *, #5608, .T. ) ;
#35840=DIRECTION ( 'NONE',  ( -0.1736481776669312471, 0.9848077530122077983, -5.551115123125779621E-17 ) ) ;
#35865=ORIENTED_EDGE ( 'NONE', *, *, #6119, .T. ) ;
#35885=CARTESIAN_POINT ( 'NONE',  ( 15.24999999999999289, 2.688986455804112996, 8.896908036367455278E-17 ) ) ;
#35955=PRESENTATION_STYLE_ASSIGNMENT (( #60327 ) ) ;
#36033=VERTEX_POINT ( 'NONE', #6238 ) ;
#36092=( NAMED_UNIT ( * ) PLANE_ANGLE_UNIT ( ) SI_UNIT ( $, .RADIAN. ) );
#36276=VERTEX_POINT ( 'NONE', #13778 ) ;
#36309=FACE_OUTER_BOUND ( 'NONE', #27857, .T. ) ;
#36331=CARTESIAN_POINT ( 'NONE',  ( 14.84250595937556483, 5.000000000000012434, -2.300655493813809945E-30 ) ) ;
#36371=AXIS2_PLACEMENT_3D ( 'NONE', #13403, #3051, #41303 ) ;
#36468=ORIENTED_EDGE ( 'NONE', *, *, #49696, .T. ) ;
#36590=CYLINDRICAL_SURFACE ( 'NONE', #7823, 9.500000000000005329 ) ;
#36669=VERTEX_POINT ( 'NONE', #4556 ) ;
#36808=ORIENTED_EDGE ( 'NONE', *, *, #50234, .T. ) ;
#36810=PLANE ( 'NONE',  #43805 ) ;
#36932=DIRECTION ( 'NONE',  ( 1.836970198721027962E-16, -1.000000000000000000, 1.069580750882383731E-61 ) ) ;
#36996=VECTOR ( 'NONE', #53002, 1000.000000000000000 ) ;
#37028=LINE ( 'NONE', #52007, #5814 ) ;
#37116=CARTESIAN_POINT ( 'NONE',  ( 16.60577576646022635, -4.999999999999987566, 6.123233995736738672E-16 ) ) ;
#37128=VERTEX_POINT ( 'NONE', #6020 ) ;
#37175=AXIS2_PLACEMENT_3D ( 'NONE', #9697, #47928, #4976 ) ;
#37313=CARTESIAN_POINT ( 'NONE',  ( -49.49999999999975842, 4.769696007084736067, -1.500000000000002220 ) ) ;
#37320=ORIENTED_EDGE ( 'NONE', *, *, #49016, .F. ) ;
#37344=EDGE_CURVE ( 'NONE', #37128, #37711, #13690, .T. ) ;
#37348=EDGE_LOOP ( 'NONE', ( #32800, #51309, #2292, #43294, #36808, #53375 ) ) ;
#37370=CARTESIAN_POINT ( 'NONE',  ( -7.955290792335435235, 8.751533712787090025, -2.059410264200305690E-15 ) ) ;
#37435=CYLINDRICAL_SURFACE ( 'NONE', #53820, 9.500000000000000000 ) ;
#37463=VERTEX_POINT ( 'NONE', #60665 ) ;
#37494=ORIENTED_EDGE ( 'NONE', *, *, #5497, .T. ) ;
#37522=VERTEX_POINT ( 'NONE', #4569 ) ;
#37524=DIRECTION ( 'NONE',  ( 0.1736481776669314414, -0.9848077530122079093, 5.551115123125779621E-17 ) ) ;
#37589=AXIS2_PLACEMENT_3D ( 'NONE', #33046, #9517, #24552 ) ;
#37630=( LENGTH_UNIT ( ) NAMED_UNIT ( * ) SI_UNIT ( .MILLI., .METRE. ) );
#37711=VERTEX_POINT ( 'NONE', #44391 ) ;
#37721=CYLINDRICAL_SURFACE ( 'NONE', #22583, 10.00000000000000711 ) ;
#37722=EDGE_LOOP ( 'NONE', ( #12840, #3726, #53778, #57855 ) ) ;
#37755=CARTESIAN_POINT ( 'NONE',  ( -6.203732170862584994, -1.182048853166489222, 5.744326400484686099E-14 ) ) ;
#37792=CARTESIAN_POINT ( 'NONE',  ( 3.173036816750036238, 10.71375812043179643, -2.686686273116197949E-15 ) ) ;
#37915=FACE_OUTER_BOUND ( 'NONE', #7872, .T. ) ;
#37981=AXIS2_PLACEMENT_3D ( 'NONE', #32535, #45720, #51614 ) ;
#38051=DIRECTION ( 'NONE',  ( -0.1736481776669312471, 0.9848077530122077983, -5.551115123125779621E-17 ) ) ;
#38324=LINE ( 'NONE', #38631, #36996 ) ;
#38501=VERTEX_POINT ( 'NONE', #29749 ) ;
#38631=CARTESIAN_POINT ( 'NONE',  ( -49.49999999999975842, 5.000000000000000000, 1.078520768856852078E-29 ) ) ;
#38668=LINE ( 'NONE', #34266, #16911 ) ;
#38677=EDGE_CURVE ( 'NONE', #55939, #37522, #26801, .T. ) ;
#38695=DIRECTION ( 'NONE',  ( -0.9848077530122077983, -0.1736481776669316079, 1.387778780781445367E-17 ) ) ;
#38846=EDGE_LOOP ( 'NONE', ( #5835, #3247, #7167, #61690, #10920 ) ) ;
#38874=CIRCLE ( 'NONE', #39864, 10.00000000000000711 ) ;
#38892=AXIS2_PLACEMENT_3D ( 'NONE', #662, #18878, #47365 ) ;
#38952=DIRECTION ( 'NONE',  ( 0.1736481776669315524, -0.9848077530122079093, 5.551115123125782702E-17 ) ) ;
#38979=EDGE_CURVE ( 'NONE', #38501, #5305, #684, .T. ) ;
#39098=FACE_BOUND ( 'NONE', #7246, .T. ) ;
#39316=DIRECTION ( 'NONE',  ( -1.836970198721033632E-16, 1.000000000000000000, 0.000000000000000000 ) ) ;
#39337=CARTESIAN_POINT ( 'NONE',  ( -16.98648177666931858, 7.159091074317976755, -1.550344604434408250E-15 ) ) ;
#39362=VECTOR ( 'NONE', #14662, 1000.000000000000114 ) ;
#39472=LINE ( 'NONE', #43247, #29896 ) ;
#39481=DIRECTION ( 'NONE',  ( -1.836970198721032153E-16, 1.000000000000000000, -1.110223024625156540E-16 ) ) ;
#39550=CARTESIAN_POINT ( 'NONE',  ( -16.98648177666932213, 7.159091074317976755, -1.550344604434408250E-15 ) ) ;
#39599=DIRECTION ( 'NONE',  ( -1.836970198721032153E-16, 1.000000000000000000, -1.110223024625156540E-16 ) ) ;
#39739=CARTESIAN_POINT ( 'NONE',  ( -99.49999999999975842, 2.999999999999992895, -1.500000000000000666 ) ) ;
#39831=DIRECTION ( 'NONE',  ( 7.985424459127866231E-16, -4.551914400963141816E-15, 1.000000000000000000 ) ) ;
#39864=AXIS2_PLACEMENT_3D ( 'NONE', #54459, #2467, #53842 ) ;
#39897=EDGE_LOOP ( 'NONE', ( #54927, #42327, #61704, #8794, #46135 ) ) ;
#39910=DIRECTION ( 'NONE',  ( 0.000000000000000000, 1.000000000000000000, 0.000000000000000000 ) ) ;
#39970=DIRECTION ( 'NONE',  ( 0.9848077530122079093, 0.1736481776669314414, -5.551115123125783935E-17 ) ) ;
#39974=DIRECTION ( 'NONE',  ( 1.000000000000000000, 1.836970198721027962E-16, -2.033782021272921061E-31 ) ) ;
#40051=FILL_AREA_STYLE ('',( #16838 ) ) ;
#40064=DIRECTION ( 'NONE',  ( 0.1736481776669314969, -0.9848077530122079093, -4.496403249731880833E-15 ) ) ;
#40443=ORIENTED_EDGE ( 'NONE', *, *, #29937, .F. ) ;
#40653=PLANE ( 'NONE',  #59536 ) ;
#40657=DIRECTION ( 'NONE',  ( 0.1736481776669316079, -0.9848077530122079093, -5.551115123125822145E-17 ) ) ;
#40694=CARTESIAN_POINT ( 'NONE',  ( -6.675040713419566174, 8.977276343754100552, -2.131574760800940707E-15 ) ) ;
#40749=DIRECTION ( 'NONE',  ( -0.9848077530122079093, -0.1736481776669314414, 5.551115123125783935E-17 ) ) ;
#40755=CARTESIAN_POINT ( 'NONE',  ( -4.923482091946712380, -0.9563062221994939049, 3.000000000000061284 ) ) ;
#40801=( LENGTH_UNIT ( ) NAMED_UNIT ( * ) SI_UNIT ( .MILLI., .METRE. ) );
#40911=ORIENTED_EDGE ( 'NONE', *, *, #3103, .F. ) ;
#40942=AXIS2_PLACEMENT_3D ( 'NONE', #43367, #15460, #39910 ) ;
#41048=EDGE_CURVE ( 'NONE', #600, #32441, #26685, .T. ) ;
#41080=CARTESIAN_POINT ( 'NONE',  ( -16.98648177666931858, 7.159091074317976755, -1.550344604434408250E-15 ) ) ;
#41200=DIRECTION ( 'NONE',  ( 1.000000000000000000, 1.836970198721027715E-16, 2.280301054154487250E-31 ) ) ;
#41303=DIRECTION ( 'NONE',  ( 0.000000000000000000, 1.000000000000000000, 0.000000000000000000 ) ) ;
#41317=CARTESIAN_POINT ( 'NONE',  ( -99.50001199999974233, 2.999999999999994671, 1.500000000000001554 ) ) ;
#41389=CARTESIAN_POINT ( 'NONE',  ( 50.50000000000024869, 1.836970198721029747E-14, -7.703719777548943412E-31 ) ) ;
#41617=CARTESIAN_POINT ( 'NONE',  ( -6.203732170862584994, -1.182048853166489222, 5.744326400484686099E-14 ) ) ;
#41706=AXIS2_PLACEMENT_3D ( 'NONE', #30038, #42933, #43868 ) ;
#41831=EDGE_CURVE ( 'NONE', #35339, #43120, #2158, .T. ) ;
#41844=ORIENTED_EDGE ( 'NONE', *, *, #5838, .F. ) ;
#42031=LINE ( 'NONE', #18205, #21022 ) ;
#42228=CARTESIAN_POINT ( 'NONE',  ( 6.189768672337906175, 1.091423221261470733, -2.362915713819767774E-16 ) ) ;
#42327=ORIENTED_EDGE ( 'NONE', *, *, #53867, .F. ) ;
#42383=CYLINDRICAL_SURFACE ( 'NONE', #57369, 10.00000000000000711 ) ;
#42577=VECTOR ( 'NONE', #39970, 1000.000000000000114 ) ;
#42617=CARTESIAN_POINT ( 'NONE',  ( -6.203732170862584994, -1.182048853166489222, 5.744326400484686099E-14 ) ) ;
#42890=DIRECTION ( 'NONE',  ( 0.1736481776669315524, -0.9848077530122079093, 5.551115123125782702E-17 ) ) ;
#42900=AXIS2_PLACEMENT_3D ( 'NONE', #48006, #57670, #5054 ) ;
#42933=DIRECTION ( 'NONE',  ( 0.9848077530122080203, 0.1736481776669315247, -2.220446049250313081E-16 ) ) ;
#43050=ORIENTED_EDGE ( 'NONE', *, *, #22179, .T. ) ;
#43054=EDGE_LOOP ( 'NONE', ( #6755, #13350, #22895, #2107, #60504, #81 ) ) ;
#43056=PLANE ( 'NONE',  #46435 ) ;
#43082=CLOSED_SHELL ( 'NONE', ( #55776, #60841, #26588, #29559, #9189, #27099, #5274, #60162, #28821, #59041, #27866, #16226, #28929, #52385, #12454, #15683, #32818, #43401, #33559, #3094, #32266, #11830, #3068, #46610, #59134, #61792, #54024, #7627, #61100 ) ) ;
#43099=EDGE_LOOP ( 'NONE', ( #25365, #28434, #43050, #44941 ) ) ;
#43107=DIRECTION ( 'NONE',  ( 0.9848077530122077983, 0.1736481776669316079, -1.387778780781445367E-17 ) ) ;
#43120=VERTEX_POINT ( 'NONE', #51563 ) ;
#43193=CARTESIAN_POINT ( 'NONE',  ( 4.909518593419350374, 0.8656805903097125610, 8.896908036367455278E-17 ) ) ;
#43247=CARTESIAN_POINT ( 'NONE',  ( -4.554074483026735898, -10.53772250678246358, 5.913403440073379425E-14 ) ) ;
#43270=ORIENTED_EDGE ( 'NONE', *, *, #7987, .F. ) ;
#43294=ORIENTED_EDGE ( 'NONE', *, *, #49696, .F. ) ;
#43300=CARTESIAN_POINT ( 'NONE',  ( 4.909518593371827500, 0.8656805903013302661, 3.058095148607754396E-16 ) ) ;
#43367=CARTESIAN_POINT ( 'NONE',  ( 50.50000000000024869, 1.836970198721029747E-14, -7.703719777548943412E-31 ) ) ;
#43401=ADVANCED_FACE ( 'NONE', ( #45293, #22083 ), #2335, .T. ) ;
#43484=CIRCLE ( 'NONE', #13470, 10.00000000000000355 ) ;
#43546=EDGE_CURVE ( 'NONE', #44582, #36033, #23621, .T. ) ;
#43581=EDGE_CURVE ( 'NONE', #24805, #600, #38668, .T. ) ;
#43586=EDGE_CURVE ( 'NONE', #52714, #7789, #24909, .T. ) ;
#43635=PRODUCT_DEFINITION ( 'UNKNOWN', '', #2860, #24815 ) ;
#43650=CARTESIAN_POINT ( 'NONE',  ( -2.700785417809981936, -13.56184546075580322, 3.000000000000003997 ) ) ;
#43805=AXIS2_PLACEMENT_3D ( 'NONE', #23309, #41200, #2948 ) ;
#43852=CIRCLE ( 'NONE', #25790, 9.499999999999996447 ) ;
#43868=DIRECTION ( 'NONE',  ( -0.1736481776669314137, 0.9848077530122077983, -5.551115123125779004E-17 ) ) ;
#43917=DIRECTION ( 'NONE',  ( 0.1736481776669315247, -0.9848077530122079093, 5.551115123125782702E-17 ) ) ;
#43930=FACE_OUTER_BOUND ( 'NONE', #4057, .T. ) ;
#43968=DIRECTION ( 'NONE',  ( 0.9848077530122077983, 0.1736481776669316079, -1.387778780781445367E-17 ) ) ;
#43978=LINE ( 'NONE', #58014, #3542 ) ;
#44108=DIRECTION ( 'NONE',  ( 0.9848077530122079093, 0.1736481776669314414, -5.551115123125783935E-17 ) ) ;
#44142=EDGE_CURVE ( 'NONE', #24192, #15612, #21942, .T. ) ;
#44234=DIRECTION ( 'NONE',  ( 0.1736481776669316079, -0.9848077530122079093, -5.551115123125822145E-17 ) ) ;
#44335=FACE_OUTER_BOUND ( 'NONE', #54157, .T. ) ;
#44361=ORIENTED_EDGE ( 'NONE', *, *, #46681, .F. ) ;
#44390=EDGE_CURVE ( 'NONE', #50838, #28664, #15894, .T. ) ;
#44391=CARTESIAN_POINT ( 'NONE',  ( 16.98648177666931502, -7.159091074317975867, -9.346835372692149838E-16 ) ) ;
#44582=VERTEX_POINT ( 'NONE', #55616 ) ;
#44665=DIRECTION ( 'NONE',  ( 0.9848077530122077983, 0.1736481776669316079, -1.387778780781445367E-17 ) ) ;
#44793=APPLICATION_CONTEXT ( 'automotive_design' ) ;
#44819=VERTEX_POINT ( 'NONE', #52005 ) ;
#44834=FACE_OUTER_BOUND ( 'NONE', #6363, .T. ) ;
#44839=EDGE_CURVE ( 'NONE', #59128, #14410, #9097, .T. ) ;
#44850=CARTESIAN_POINT ( 'NONE',  ( -6.203732170862584994, -1.182048853166489222, 5.744326400484686099E-14 ) ) ;
#44857=DIRECTION ( 'NONE',  ( 0.000000000000000000, 1.000000000000000000, 0.000000000000000000 ) ) ;
#44941=ORIENTED_EDGE ( 'NONE', *, *, #47160, .F. ) ;
#44944=FACE_OUTER_BOUND ( 'NONE', #43099, .T. ) ;
#45002=ORIENTED_EDGE ( 'NONE', *, *, #37344, .F. ) ;
#45051=SURFACE_SIDE_STYLE ('',( #3316 ) ) ;
#45156=EDGE_CURVE ( 'NONE', #55623, #28664, #18437, .T. ) ;
#45159=ORIENTED_EDGE ( 'NONE', *, *, #49753, .F. ) ;
#45190=AXIS2_PLACEMENT_3D ( 'NONE', #29418, #19729, #33838 ) ;
#45267=AXIS2_PLACEMENT_3D ( 'NONE', #5130, #38695, #27495 ) ;
#45293=FACE_BOUND ( 'NONE', #3012, .T. ) ;
#45372=VECTOR ( 'NONE', #15567, 1000.000000000000000 ) ;
#45480=VERTEX_POINT ( 'NONE', #51235 ) ;
#45720=DIRECTION ( 'NONE',  ( 0.9848077530122080203, 0.1736481776669314692, -5.551115123125783935E-17 ) ) ;
#45757=AXIS2_PLACEMENT_3D ( 'NONE', #12147, #1775, #40657 ) ;
#45783=LINE ( 'NONE', #60152, #25042 ) ;
#45940=CIRCLE ( 'NONE', #42900, 5.000000000000000000 ) ;
#45949=ORIENTED_EDGE ( 'NONE', *, *, #4066, .T. ) ;
#45990=ORIENTED_EDGE ( 'NONE', *, *, #17137, .F. ) ;
#46104=VERTEX_POINT ( 'NONE', #9111 ) ;
#46107=SURFACE_SIDE_STYLE ('',( #51694 ) ) ;
#46135=ORIENTED_EDGE ( 'NONE', *, *, #60258, .T. ) ;
#46219=CARTESIAN_POINT ( 'NONE',  ( -2.700785417809989042, -13.56184546075576769, -3.000000000000003997 ) ) ;
#46220=( BOUNDED_CURVE ( )  B_SPLINE_CURVE ( 3, ( #61652, #30938, #49732, #31245 ),
 .UNSPECIFIED., .F., .F. ) 
 B_SPLINE_CURVE_WITH_KNOTS ( ( 4, 4 ),
 ( 3.141592653589793116, 6.283185307179586232 ),
 .UNSPECIFIED. ) 
 CURVE ( )  GEOMETRIC_REPRESENTATION_ITEM ( )  RATIONAL_B_SPLINE_CURVE ( ( 1.000000000000000000, 0.3333333333333333703, 0.3333333333333333703, 1.000000000000000000 ) ) 
 REPRESENTATION_ITEM ( '' )  );
#46435=AXIS2_PLACEMENT_3D ( 'NONE', #58644, #15771, #28928 ) ;
#46438=ORIENTED_EDGE ( 'NONE', *, *, #33336, .F. ) ;
#46538=SHAPE_DEFINITION_REPRESENTATION ( #19921, #27649 ) ;
#46560=AXIS2_PLACEMENT_3D ( 'NONE', #10651, #5596, #57922 ) ;
#46610=ADVANCED_FACE ( 'NONE', ( #8261 ), #36810, .F. ) ;
#46681=EDGE_CURVE ( 'NONE', #12966, #43120, #28609, .T. ) ;
#46718=PRESENTATION_STYLE_ASSIGNMENT (( #12897 ) ) ;
#46866=ORIENTED_EDGE ( 'NONE', *, *, #53867, .T. ) ;
#47160=EDGE_CURVE ( 'NONE', #46104, #5234, #17747, .T. ) ;
#47230=AXIS2_PLACEMENT_3D ( 'NONE', #58156, #15277, #209 ) ;
#47322=DIRECTION ( 'NONE',  ( 8.032841876251139751E-16, -4.551914400963141816E-15, 1.000000000000000000 ) ) ;
#47340=CARTESIAN_POINT ( 'NONE',  ( 4.909518593422035337, 0.8656805902944597619, 8.896908036367455278E-17 ) ) ;
#47365=DIRECTION ( 'NONE',  ( -0.9848077530122077983, -0.1736481776669316079, 1.387778780781445367E-17 ) ) ;
#47390=AXIS2_PLACEMENT_3D ( 'NONE', #44850, #11308, #25711 ) ;
#47424=DIRECTION ( 'NONE',  ( 2.280301054154487250E-31, 0.000000000000000000, -1.000000000000000000 ) ) ;
#47460=EDGE_CURVE ( 'NONE', #36276, #24805, #20789, .T. ) ;
#47475=CIRCLE ( 'NONE', #6421, 10.00000000000000711 ) ;
#47483=CARTESIAN_POINT ( 'NONE',  ( 6.189768672335216770, 1.091423221276722755, -1.945113688487589062E-17 ) ) ;
#47492=FACE_OUTER_BOUND ( 'NONE', #37348, .T. ) ;
#47614=DIRECTION ( 'NONE',  ( 0.1736481776669314414, -0.9848077530122079093, 5.551115123125779004E-17 ) ) ;
#47715=CARTESIAN_POINT ( 'NONE',  ( -15.25000000000000711, -2.688986455804108555, -9.952330921218299798E-16 ) ) ;
#47775=ORIENTED_EDGE ( 'NONE', *, *, #51689, .F. ) ;
#47928=DIRECTION ( 'NONE',  ( -0.9848077530122080203, -0.1736481776669315524, 2.220446049250313574E-16 ) ) ;
#48006=CARTESIAN_POINT ( 'NONE',  ( -99.49999999999975842, -9.184850993605117179E-15, 3.081487911019577365E-29 ) ) ;
#48029=ORIENTED_EDGE ( 'NONE', *, *, #48278, .T. ) ;
#48131=ORIENTED_EDGE ( 'NONE', *, *, #50356, .T. ) ;
#48253=ORIENTED_EDGE ( 'NONE', *, *, #17141, .T. ) ;
#48278=EDGE_CURVE ( 'NONE', #44819, #36669, #43852, .T. ) ;
#48353=CARTESIAN_POINT ( 'NONE',  ( -13.51351822333069030, -12.53706398592619387, 7.845252193381024343E-16 ) ) ;
#48383=DIRECTION ( 'NONE',  ( -0.9848077530122077983, -0.1736481776669315802, 5.551115123125782702E-17 ) ) ;
#48460=LINE ( 'NONE', #19665, #39362 ) ;
#48624=DIRECTION ( 'NONE',  ( 0.9848077530122079093, 0.1736481776669316079, -5.551115123125783935E-17 ) ) ;
#48633=AXIS2_PLACEMENT_3D ( 'NONE', #49026, #39974, #58705 ) ;
#48711=LINE ( 'NONE', #39337, #42577 ) ;
#48864=ORIENTED_EDGE ( 'NONE', *, *, #1209, .F. ) ;
#48957=ORIENTED_EDGE ( 'NONE', *, *, #12842, .T. ) ;
#49016=EDGE_CURVE ( 'NONE', #16043, #12966, #27725, .T. ) ;
#49026=CARTESIAN_POINT ( 'NONE',  ( -49.49999999999975842, 1.232595164407830946E-29, 1.078520768856852078E-29 ) ) ;
#49149=ORIENTED_EDGE ( 'NONE', *, *, #8921, .F. ) ;
#49325=FACE_OUTER_BOUND ( 'NONE', #43054, .T. ) ;
#49377=CARTESIAN_POINT ( 'NONE',  ( -16.98648177666931858, 7.159091074317976755, -1.550344604434408250E-15 ) ) ;
#49616=AXIS2_PLACEMENT_3D ( 'NONE', #52717, #52097, #38051 ) ;
#49659=AXIS2_PLACEMENT_3D ( 'NONE', #34739, #54420, #1495 ) ;
#49663=STYLED_ITEM ( 'NONE', ( #46718 ), #51224 ) ;
#49696=EDGE_CURVE ( 'NONE', #32441, #58934, #27849, .T. ) ;
#49710=EDGE_LOOP ( 'NONE', ( #60732, #6061, #45002, #9732 ) ) ;
#49732=CARTESIAN_POINT ( 'NONE',  ( 16.60577576646022280, -4.999999999999991118, -10.00000000000000711 ) ) ;
#49753=EDGE_CURVE ( 'NONE', #58934, #43120, #24652, .T. ) ;
#50234=EDGE_CURVE ( 'NONE', #32441, #37522, #30186, .T. ) ;
#50241=DIRECTION ( 'NONE',  ( -0.1736481776669312471, 0.9848077530122077983, -5.551115123125779621E-17 ) ) ;
#50356=EDGE_CURVE ( 'NONE', #21914, #44582, #6266, .T. ) ;
#50554=VECTOR ( 'NONE', #39481, 1000.000000000000000 ) ;
#50682=COLOUR_RGB ( '', 0.40784314, 0.44705882, 0.49803922) ;
#50707=EDGE_CURVE ( 'NONE', #61564, #15612, #2304, .T. ) ;
#50757=AXIS2_PLACEMENT_3D ( 'NONE', #41317, #36932, #55995 ) ;
#50787=APPLICATION_CONTEXT ( 'automotive_design' ) ;
#50838=VERTEX_POINT ( 'NONE', #546 ) ;
#50939=( NAMED_UNIT ( * ) PLANE_ANGLE_UNIT ( ) SI_UNIT ( $, .RADIAN. ) );
#50969=FACE_OUTER_BOUND ( 'NONE', #7388, .T. ) ;
#51018=MANIFOLD_SOLID_BREP ( 'Cut-Extrude-Thin4', #43082 ) ;
#51074=( NAMED_UNIT ( * ) PLANE_ANGLE_UNIT ( ) SI_UNIT ( $, .RADIAN. ) );
#51224=ADVANCED_BREP_SHAPE_REPRESENTATION ( '', ( #51018, #14677 ), #15707 ) ;
#51235=CARTESIAN_POINT ( 'NONE',  ( 4.453286895665903522, 10.93950075139880518, -2.758850769716832966E-15 ) ) ;
#51309=ORIENTED_EDGE ( 'NONE', *, *, #3667, .F. ) ;
#51456=DIRECTION ( 'NONE',  ( -0.9848077530122077983, -0.1736481776669316079, 1.387778780781445367E-17 ) ) ;
#51465=VERTEX_POINT ( 'NONE', #37116 ) ;
#51563=CARTESIAN_POINT ( 'NONE',  ( -79.49999999999975842, 2.999999999999995559, -1.499999999999999778 ) ) ;
#51614=DIRECTION ( 'NONE',  ( -0.1736481776669312471, 0.9848077530122077983, -5.551115123125779621E-17 ) ) ;
#51644=EDGE_LOOP ( 'NONE', ( #9464, #12222, #45159, #32370 ) ) ;
#51689=EDGE_CURVE ( 'NONE', #55623, #11621, #31624, .T. ) ;
#51694=SURFACE_STYLE_FILL_AREA ( #22591 ) ;
#51760=VECTOR ( 'NONE', #5613, 1000.000000000000000 ) ;
#51896=EDGE_CURVE ( 'NONE', #61564, #50838, #16222, .T. ) ;
#51920=AXIS2_PLACEMENT_3D ( 'NONE', #5426, #30472, #33979 ) ;
#52005=CARTESIAN_POINT ( 'NONE',  ( -3.273824404110865061, -10.31197987581545306, 5.906186990413314898E-14 ) ) ;
#52007=CARTESIAN_POINT ( 'NONE',  ( -13.59350196068899841, -12.08345367038093521, -2.999999999999984013 ) ) ;
#52017=EDGE_LOOP ( 'NONE', ( #8549, #45949, #48029, #54103 ) ) ;
#52097=DIRECTION ( 'NONE',  ( 0.9848077530122080203, 0.1736481776669314692, -5.551115123125783935E-17 ) ) ;
#52132=CARTESIAN_POINT ( 'NONE',  ( -99.50001199999974233, 2.999999999999994671, 1.500000000000001554 ) ) ;
#52166=ORIENTED_EDGE ( 'NONE', *, *, #43586, .F. ) ;
#52216=DIRECTION ( 'NONE',  ( 0.000000000000000000, 1.000000000000000000, 0.000000000000000000 ) ) ;
#52303=PLANE ( 'NONE',  #17530 ) ;
#52358=FACE_OUTER_BOUND ( 'NONE', #18371, .T. ) ;
#52385=ADVANCED_FACE ( 'NONE', ( #6320, #25149 ), #43056, .T. ) ;
#52478=DIRECTION ( 'NONE',  ( 0.000000000000000000, 1.000000000000000000, 0.000000000000000000 ) ) ;
#52507=EDGE_LOOP ( 'NONE', ( #60640, #9743 ) ) ;
#52714=VERTEX_POINT ( 'NONE', #57642 ) ;
#52717=CARTESIAN_POINT ( 'NONE',  ( -15.25000000000000711, -2.688986455804108555, -9.952330921218299798E-16 ) ) ;
#52943=ORIENTED_EDGE ( 'NONE', *, *, #43581, .T. ) ;
#52949=DIRECTION ( 'NONE',  ( -0.9848077530122077983, -0.1736481776669316079, 1.387778780781445367E-17 ) ) ;
#53002=DIRECTION ( 'NONE',  ( 1.000000000000000000, 1.836970198721027962E-16, -2.033782021272921061E-31 ) ) ;
#53042=FACE_OUTER_BOUND ( 'NONE', #52017, .T. ) ;
#53072=CARTESIAN_POINT ( 'NONE',  ( 6.189768672337906175, 1.091423221261470733, -2.362915713819767774E-16 ) ) ;
#53081=EDGE_CURVE ( 'NONE', #59128, #50838, #2340, .T. ) ;
#53218=PLANE ( 'NONE',  #45190 ) ;
#53341=DIRECTION ( 'NONE',  ( 0.9848077530122079093, 0.1736481776669314414, -5.551115123125783935E-17 ) ) ;
#53375=ORIENTED_EDGE ( 'NONE', *, *, #1209, .T. ) ;
#53415=ORIENTED_EDGE ( 'NONE', *, *, #14867, .T. ) ;
#53533=CARTESIAN_POINT ( 'NONE',  ( -4.923482091946717709, -0.9563062221994661494, -2.999999999999945377 ) ) ;
#53778=ORIENTED_EDGE ( 'NONE', *, *, #7987, .T. ) ;
#53820=AXIS2_PLACEMENT_3D ( 'NONE', #37755, #32727, #5414 ) ;
#53842=DIRECTION ( 'NONE',  ( 0.1736481776669314137, -0.9848077530122077983, 5.551115123125779621E-17 ) ) ;
#53867=EDGE_CURVE ( 'NONE', #11621, #14410, #12439, .T. ) ;
#54024=ADVANCED_FACE ( 'NONE', ( #47492 ), #4540, .T. ) ;
#54103=ORIENTED_EDGE ( 'NONE', *, *, #12842, .F. ) ;
#54157=EDGE_LOOP ( 'NONE', ( #23585, #18143 ) ) ;
#54175=DIRECTION ( 'NONE',  ( -0.9848077530122077983, -0.1736481776669316079, 1.387778780781445367E-17 ) ) ;
#54224=ORIENTED_EDGE ( 'NONE', *, *, #22179, .F. ) ;
#54420=DIRECTION ( 'NONE',  ( 0.9848077530122080203, 0.1736481776669315247, -2.220446049250313081E-16 ) ) ;
#54459=CARTESIAN_POINT ( 'NONE',  ( -6.218809015666120210, -1.096543817334992621, 4.142297321093258830E-16 ) ) ;
#54498=DIRECTION ( 'NONE',  ( -0.9848077530122080203, -0.1736481776669315524, 2.220446049250313574E-16 ) ) ;
#54695=ORIENTED_EDGE ( 'NONE', *, *, #7323, .F. ) ;
#54757=CARTESIAN_POINT ( 'NONE',  ( -6.218809015666120210, -1.096543817334992621, 4.142297321093258830E-16 ) ) ;
#54779=CARTESIAN_POINT ( 'NONE',  ( 4.909518593419350374, 0.8656805903097125610, 8.896908036367455278E-17 ) ) ;
#54882=AXIS2_PLACEMENT_3D ( 'NONE', #35885, #54955, #12089 ) ;
#54925=CARTESIAN_POINT ( 'NONE',  ( -15.25000000000000711, -2.688986455804108555, -9.952330921218299798E-16 ) ) ;
#54927=ORIENTED_EDGE ( 'NONE', *, *, #44839, .T. ) ;
#54955=DIRECTION ( 'NONE',  ( 0.9848077530122079093, 0.1736481776669314137, -2.220446049250313081E-16 ) ) ;
#55095=VERTEX_POINT ( 'NONE', #33955 ) ;
#55135=DIRECTION ( 'NONE',  ( 1.000000000000000000, 1.836970198721027715E-16, -2.218671295934095703E-31 ) ) ;
#55238=AXIS2_PLACEMENT_3D ( 'NONE', #47340, #52949, #33259 ) ;
#55448=DIRECTION ( 'NONE',  ( 1.000000000000000000, 1.836970198721027962E-16, -2.033782021272921061E-31 ) ) ;
#55576=DIRECTION ( 'NONE',  ( 0.9848077530122079093, 0.1736481776669316079, -5.551115123125783935E-17 ) ) ;
#55616=CARTESIAN_POINT ( 'NONE',  ( -13.51351822333069030, -12.53706398592619387, 7.845252193381024343E-16 ) ) ;
#55623=VERTEX_POINT ( 'NONE', #29164 ) ;
#55629=( LENGTH_UNIT ( ) NAMED_UNIT ( * ) SI_UNIT ( .MILLI., .METRE. ) );
#55776=ADVANCED_FACE ( 'NONE', ( #37915 ), #27556, .T. ) ;
#55939=VERTEX_POINT ( 'NONE', #26236 ) ;
#55976=DIRECTION ( 'NONE',  ( -0.9848077530122077983, -0.1736481776669315802, 5.551115123125782702E-17 ) ) ;
#55995=DIRECTION ( 'NONE',  ( 1.000000000000000000, 1.836970198721027962E-16, -2.033782021272921061E-31 ) ) ;
#56127=EDGE_CURVE ( 'NONE', #15021, #24192, #24549, .T. ) ;
#56201=EDGE_CURVE ( 'NONE', #16043, #24805, #30464, .T. ) ;
#56323=EDGE_LOOP ( 'NONE', ( #41844, #59564, #11337, #760 ) ) ;
#56389=DIRECTION ( 'NONE',  ( 1.836970198721031906E-16, -1.000000000000000000, 1.110223024625156540E-16 ) ) ;
#56883=ORIENTED_EDGE ( 'NONE', *, *, #8921, .T. ) ;
#56942=VECTOR ( 'NONE', #6883, 1000.000000000000114 ) ;
#57257=ORIENTED_EDGE ( 'NONE', *, *, #6119, .F. ) ;
#57283=FACE_OUTER_BOUND ( 'NONE', #19051, .T. ) ;
#57307=EDGE_CURVE ( 'NONE', #5305, #38501, #31517, .T. ) ;
#57369=AXIS2_PLACEMENT_3D ( 'NONE', #23556, #23872, #28254 ) ;
#57525=( BOUNDED_CURVE ( )  B_SPLINE_CURVE ( 3, ( #16, #34179, #18852, #24450 ),
 .UNSPECIFIED., .F., .F. ) 
 B_SPLINE_CURVE_WITH_KNOTS ( ( 4, 4 ),
 ( 0.000000000000000000, 3.141592653589793116 ),
 .UNSPECIFIED. ) 
 CURVE ( )  GEOMETRIC_REPRESENTATION_ITEM ( )  RATIONAL_B_SPLINE_CURVE ( ( 1.000000000000000000, 0.3333333333333333703, 0.3333333333333333703, 1.000000000000000000 ) ) 
 REPRESENTATION_ITEM ( '' )  );
#57551=AXIS2_PLACEMENT_3D ( 'NONE', #54779, #43968, #38952 ) ;
#57556=VECTOR ( 'NONE', #29826, 1000.000000000000000 ) ;
#57586=EDGE_CURVE ( 'NONE', #45480, #37128, #11483, .T. ) ;
#57642=CARTESIAN_POINT ( 'NONE',  ( 50.50000000000024869, 5.000000000000018652, -7.703719777548943412E-31 ) ) ;
#57644=AXIS2_PLACEMENT_3D ( 'NONE', #34957, #30228, #25844 ) ;
#57670=DIRECTION ( 'NONE',  ( -1.000000000000000000, -1.836970198721027715E-16, 2.218671295934095703E-31 ) ) ;
#57855=ORIENTED_EDGE ( 'NONE', *, *, #20975, .F. ) ;
#57922=DIRECTION ( 'NONE',  ( 2.218671295934095703E-31, -1.000000000000000000, 1.110223024625156540E-16 ) ) ;
#58007=LINE ( 'NONE', #15131, #57556 ) ;
#58014=CARTESIAN_POINT ( 'NONE',  ( -13.51351822333069030, -12.53706398592619387, 7.845252193381024343E-16 ) ) ;
#58108=ORIENTED_EDGE ( 'NONE', *, *, #7323, .T. ) ;
#58141=ORIENTED_EDGE ( 'NONE', *, *, #56127, .T. ) ;
#58156=CARTESIAN_POINT ( 'NONE',  ( -4.938558936750251149, -0.8708011863679868680, 8.896908036367455278E-17 ) ) ;
#58220=DIRECTION ( 'NONE',  ( 0.9848077530122079093, 0.1736481776669315524, -5.551115123125781470E-17 ) ) ;
#58242=CARTESIAN_POINT ( 'NONE',  ( -99.50001199999974233, 2.999999999999992895, -1.500000000000000666 ) ) ;
#58375=STYLED_ITEM ( 'NONE', ( #35955 ), #51018 ) ;
#58376=CARTESIAN_POINT ( 'NONE',  ( 50.50000000000024869, 1.836970198721029747E-14, -7.703719777548943412E-31 ) ) ;
#58538=DIRECTION ( 'NONE',  ( 7.985424459127866231E-16, -4.551914400963141816E-15, 1.000000000000000000 ) ) ;
#58644=CARTESIAN_POINT ( 'NONE',  ( 6.189768672337906175, 1.091423221261470733, -2.362915713819767774E-16 ) ) ;
#58684=DIRECTION ( 'NONE',  ( 1.000000000000000000, 1.836970198721033632E-16, -2.218671295934095703E-31 ) ) ;
#58705=DIRECTION ( 'NONE',  ( 0.000000000000000000, 1.000000000000000000, 0.000000000000000000 ) ) ;
#58934=VERTEX_POINT ( 'NONE', #27285 ) ;
#59041=ADVANCED_FACE ( 'NONE', ( #24742 ), #52303, .F. ) ;
#59128=VERTEX_POINT ( 'NONE', #20360 ) ;
#59134=ADVANCED_FACE ( 'NONE', ( #25051 ), #29739, .T. ) ;
#59161=EDGE_CURVE ( 'NONE', #35339, #55095, #10032, .T. ) ;
#59265=CARTESIAN_POINT ( 'NONE',  ( -49.49999999999975842, 1.232595164407830946E-29, 1.078520768856852078E-29 ) ) ;
#59397=DIRECTION ( 'NONE',  ( 0.000000000000000000, 1.000000000000000000, -3.552713678800500929E-15 ) ) ;
#59536=AXIS2_PLACEMENT_3D ( 'NONE', #26519, #26206, #1460 ) ;
#59544=CARTESIAN_POINT ( 'NONE',  ( -7.853389858698435866, 8.173624800449486472, 5.691590806814991163E-14 ) ) ;
#59564=ORIENTED_EDGE ( 'NONE', *, *, #51896, .T. ) ;
#59797=EDGE_CURVE ( 'NONE', #45480, #37463, #12627, .T. ) ;
#59854=ORIENTED_EDGE ( 'NONE', *, *, #44390, .F. ) ;
#60120=CARTESIAN_POINT ( 'NONE',  ( -13.59350196068900196, -12.08345367038092810, 3.000000000000023981 ) ) ;
#60152=CARTESIAN_POINT ( 'NONE',  ( -49.49999999999975842, -5.000000000000000000, 6.123233995736873765E-16 ) ) ;
#60162=ADVANCED_FACE ( 'NONE', ( #19523 ), #37721, .T. ) ;
#60258=EDGE_CURVE ( 'NONE', #15021, #59128, #58007, .T. ) ;
#60322=CARTESIAN_POINT ( 'NONE',  ( 50.50000000000024869, -4.999999999999982236, 6.123233995736707118E-16 ) ) ;
#60327=SURFACE_STYLE_USAGE ( .BOTH. , #45051 ) ;
#60504=ORIENTED_EDGE ( 'NONE', *, *, #41048, .F. ) ;
#60605=ORIENTED_EDGE ( 'NONE', *, *, #51689, .T. ) ;
#60640=ORIENTED_EDGE ( 'NONE', *, *, #38979, .T. ) ;
#60665=CARTESIAN_POINT ( 'NONE',  ( 7.926250449004538012, -8.756654308845361001, -4.239809459443226272E-16 ) ) ;
#60732=ORIENTED_EDGE ( 'NONE', *, *, #59797, .T. ) ;
#60838=CARTESIAN_POINT ( 'NONE',  ( -2.700785417809981936, -13.56184546075580322, 3.000000000000003997 ) ) ;
#60841=ADVANCED_FACE ( 'NONE', ( #49325 ), #10824, .T. ) ;
#61100=ADVANCED_FACE ( 'NONE', ( #15141 ), #34248, .T. ) ;
#61352=CARTESIAN_POINT ( 'NONE',  ( -15.25000000000000711, -2.688986455804108555, -9.952330921218299798E-16 ) ) ;
#61387=DIRECTION ( 'NONE',  ( 0.000000000000000000, 0.000000000000000000, 1.000000000000000000 ) ) ;
#61395=ORIENTED_EDGE ( 'NONE', *, *, #50707, .F. ) ;
#61399=CARTESIAN_POINT ( 'NONE',  ( -14.84250595937556483, -4.999999999999993783, 6.123233995736803753E-16 ) ) ;
#61564=VERTEX_POINT ( 'NONE', #22236 ) ;
#61652=CARTESIAN_POINT ( 'NONE',  ( 14.84250595937556483, 5.000000000000012434, -2.300655493813809945E-30 ) ) ;
#61657=DIRECTION ( 'NONE',  ( 0.000000000000000000, -1.000000000000000000, 0.000000000000000000 ) ) ;
#61677=DIRECTION ( 'NONE',  ( -0.9848077530122079093, -0.1736481776669314414, 2.220446049250313081E-16 ) ) ;
#61690=ORIENTED_EDGE ( 'NONE', *, *, #47460, .T. ) ;
#61704=ORIENTED_EDGE ( 'NONE', *, *, #20971, .F. ) ;
#61792=ADVANCED_FACE ( 'NONE', ( #6089 ), #15843, .T. ) ;
#61908=DIRECTION ( 'NONE',  ( -1.000000000000000000, -1.836970198721027715E-16, 2.218671295934095703E-31 ) ) ;
ENDSEC;
END-ISO-10303-21;
